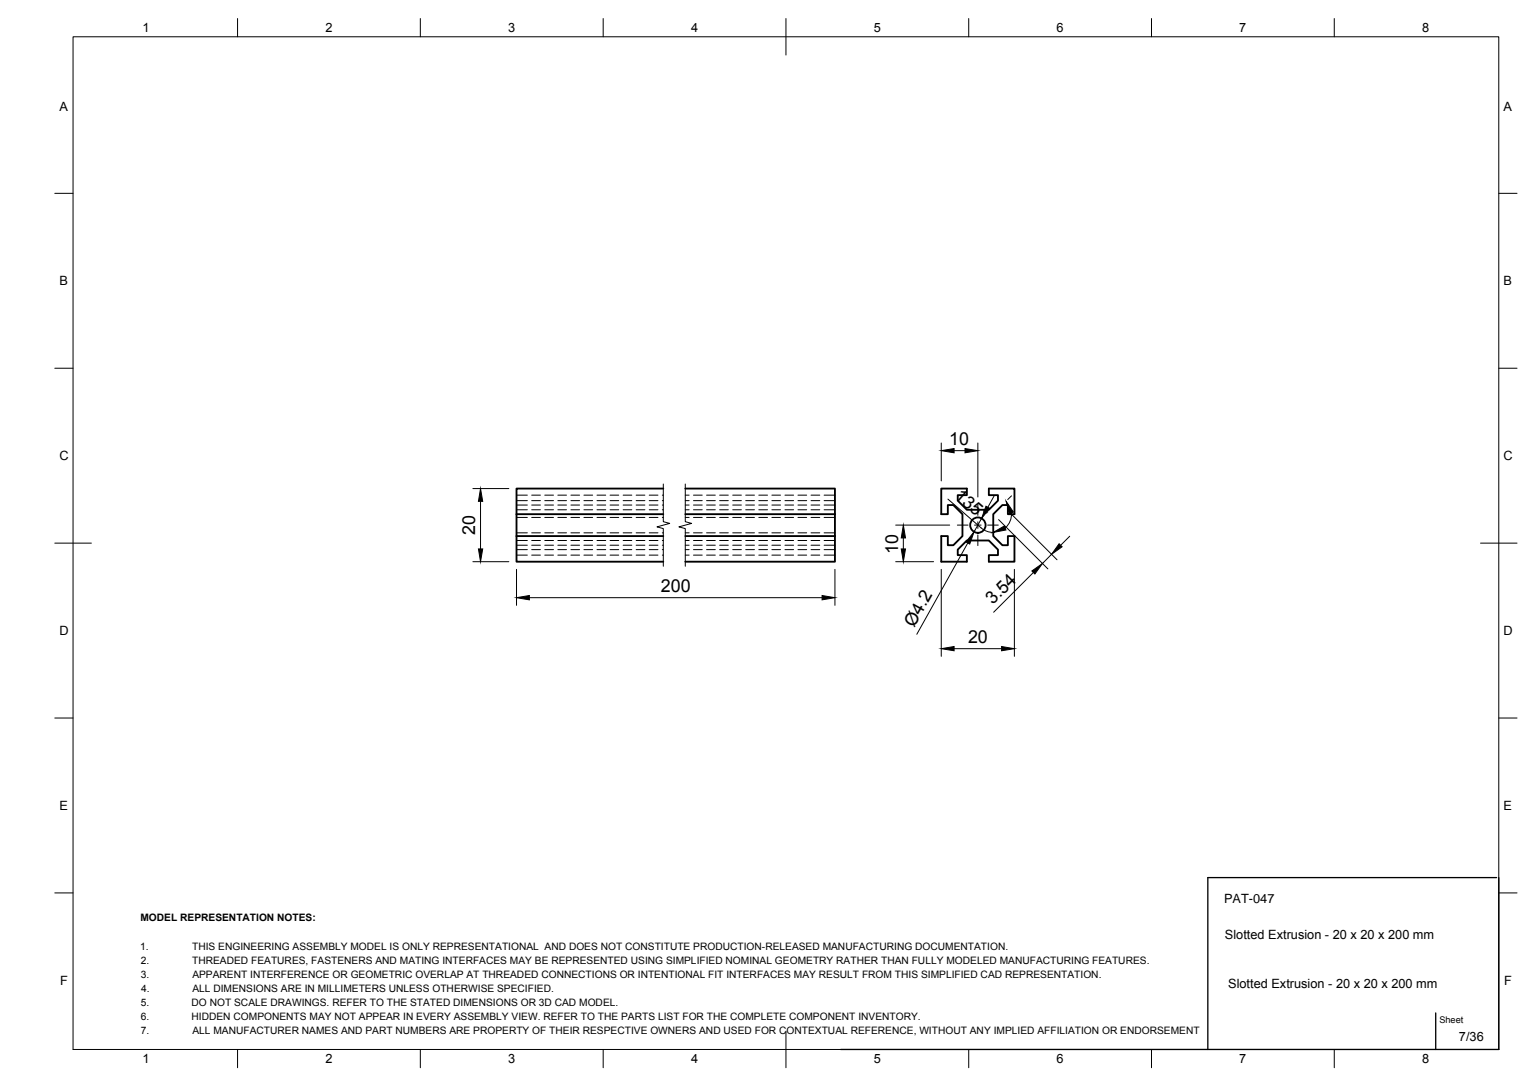
ISO-10303-21;
HEADER;
/* Generated by software containing ST-Developer
 * from STEP Tools, Inc. (www.steptools.com) 
 */

FILE_DESCRIPTION(
/* description */ ('Gravity roller conveyor section'),
/* implementation_level */ '2;1');

FILE_NAME(
/* name */ 'Slotted Extrusion - 20 x 20 x 200 mm.step',
/* time_stamp */ '2026-11-02T07:43:02-08:00',
/* author */ (''),
/* organization */ (''),
/* preprocessor_version */ 'ST-DEVELOPER v20.2',
/* originating_system */ 'Autodesk Translation Framework v15.17.0.0',
/* authorisation */ '');

FILE_SCHEMA (('AUTOMOTIVE_DESIGN { 1 0 10303 214 3 1 1 }'));
ENDSEC;

DATA;
#10=MECHANICAL_DESIGN_GEOMETRIC_PRESENTATION_REPRESENTATION('',(#532),#13821);
#464=SHAPE_REPRESENTATION_RELATIONSHIP('SRR','None',#14001,#498);
#498=ADVANCED_BREP_SHAPE_REPRESENTATION('',(#574),#13788);
#532=STYLED_ITEM('',(#14192),#574);
#574=MANIFOLD_SOLID_BREP('Body1',#7630);
#627=FACE_BOUND('',#1598,.T.);
#628=FACE_BOUND('',#1600,.T.);
#800=PLANE('',#8178);
#801=PLANE('',#8179);
#802=PLANE('',#8180);
#803=PLANE('',#8181);
#804=PLANE('',#8182);
#805=PLANE('',#8183);
#806=PLANE('',#8184);
#807=PLANE('',#8185);
#808=PLANE('',#8186);
#809=PLANE('',#8187);
#810=PLANE('',#8188);
#811=PLANE('',#8189);
#812=PLANE('',#8190);
#813=PLANE('',#8191);
#814=PLANE('',#8192);
#815=PLANE('',#8193);
#816=PLANE('',#8194);
#817=PLANE('',#8195);
#818=PLANE('',#8196);
#819=PLANE('',#8197);
#820=PLANE('',#8198);
#821=PLANE('',#8199);
#822=PLANE('',#8200);
#823=PLANE('',#8201);
#824=PLANE('',#8202);
#825=PLANE('',#8203);
#826=PLANE('',#8204);
#827=PLANE('',#8205);
#828=PLANE('',#8206);
#829=PLANE('',#8207);
#830=PLANE('',#8208);
#831=PLANE('',#8209);
#832=PLANE('',#8210);
#833=PLANE('',#8211);
#834=PLANE('',#8212);
#835=PLANE('',#8213);
#836=PLANE('',#8217);
#837=PLANE('',#8218);
#838=PLANE('',#8219);
#839=PLANE('',#8220);
#840=PLANE('',#8221);
#841=PLANE('',#8222);
#842=PLANE('',#8223);
#843=PLANE('',#8224);
#844=PLANE('',#8225);
#845=PLANE('',#8226);
#1115=FACE_OUTER_BOUND('',#1552,.T.);
#1116=FACE_OUTER_BOUND('',#1553,.T.);
#1117=FACE_OUTER_BOUND('',#1554,.T.);
#1118=FACE_OUTER_BOUND('',#1555,.T.);
#1119=FACE_OUTER_BOUND('',#1556,.T.);
#1120=FACE_OUTER_BOUND('',#1557,.T.);
#1121=FACE_OUTER_BOUND('',#1558,.T.);
#1122=FACE_OUTER_BOUND('',#1559,.T.);
#1123=FACE_OUTER_BOUND('',#1560,.T.);
#1124=FACE_OUTER_BOUND('',#1561,.T.);
#1125=FACE_OUTER_BOUND('',#1562,.T.);
#1126=FACE_OUTER_BOUND('',#1563,.T.);
#1127=FACE_OUTER_BOUND('',#1564,.T.);
#1128=FACE_OUTER_BOUND('',#1565,.T.);
#1129=FACE_OUTER_BOUND('',#1566,.T.);
#1130=FACE_OUTER_BOUND('',#1567,.T.);
#1131=FACE_OUTER_BOUND('',#1568,.T.);
#1132=FACE_OUTER_BOUND('',#1569,.T.);
#1133=FACE_OUTER_BOUND('',#1570,.T.);
#1134=FACE_OUTER_BOUND('',#1571,.T.);
#1135=FACE_OUTER_BOUND('',#1572,.T.);
#1136=FACE_OUTER_BOUND('',#1573,.T.);
#1137=FACE_OUTER_BOUND('',#1574,.T.);
#1138=FACE_OUTER_BOUND('',#1575,.T.);
#1139=FACE_OUTER_BOUND('',#1576,.T.);
#1140=FACE_OUTER_BOUND('',#1577,.T.);
#1141=FACE_OUTER_BOUND('',#1578,.T.);
#1142=FACE_OUTER_BOUND('',#1579,.T.);
#1143=FACE_OUTER_BOUND('',#1580,.T.);
#1144=FACE_OUTER_BOUND('',#1581,.T.);
#1145=FACE_OUTER_BOUND('',#1582,.T.);
#1146=FACE_OUTER_BOUND('',#1583,.T.);
#1147=FACE_OUTER_BOUND('',#1584,.T.);
#1148=FACE_OUTER_BOUND('',#1585,.T.);
#1149=FACE_OUTER_BOUND('',#1586,.T.);
#1150=FACE_OUTER_BOUND('',#1587,.T.);
#1151=FACE_OUTER_BOUND('',#1588,.T.);
#1152=FACE_OUTER_BOUND('',#1589,.T.);
#1153=FACE_OUTER_BOUND('',#1590,.T.);
#1154=FACE_OUTER_BOUND('',#1591,.T.);
#1155=FACE_OUTER_BOUND('',#1592,.T.);
#1156=FACE_OUTER_BOUND('',#1593,.T.);
#1157=FACE_OUTER_BOUND('',#1594,.T.);
#1158=FACE_OUTER_BOUND('',#1595,.T.);
#1159=FACE_OUTER_BOUND('',#1596,.T.);
#1160=FACE_OUTER_BOUND('',#1597,.T.);
#1161=FACE_OUTER_BOUND('',#1599,.T.);
#1552=EDGE_LOOP('',(#5830,#5831,#5832,#5833));
#1553=EDGE_LOOP('',(#5834,#5835,#5836,#5837));
#1554=EDGE_LOOP('',(#5838,#5839,#5840,#5841));
#1555=EDGE_LOOP('',(#5842,#5843,#5844,#5845));
#1556=EDGE_LOOP('',(#5846,#5847,#5848,#5849));
#1557=EDGE_LOOP('',(#5850,#5851,#5852,#5853));
#1558=EDGE_LOOP('',(#5854,#5855,#5856,#5857));
#1559=EDGE_LOOP('',(#5858,#5859,#5860,#5861));
#1560=EDGE_LOOP('',(#5862,#5863,#5864,#5865));
#1561=EDGE_LOOP('',(#5866,#5867,#5868,#5869));
#1562=EDGE_LOOP('',(#5870,#5871,#5872,#5873));
#1563=EDGE_LOOP('',(#5874,#5875,#5876,#5877));
#1564=EDGE_LOOP('',(#5878,#5879,#5880,#5881));
#1565=EDGE_LOOP('',(#5882,#5883,#5884,#5885));
#1566=EDGE_LOOP('',(#5886,#5887,#5888,#5889));
#1567=EDGE_LOOP('',(#5890,#5891,#5892,#5893));
#1568=EDGE_LOOP('',(#5894,#5895,#5896,#5897));
#1569=EDGE_LOOP('',(#5898,#5899,#5900,#5901));
#1570=EDGE_LOOP('',(#5902,#5903,#5904,#5905));
#1571=EDGE_LOOP('',(#5906,#5907,#5908,#5909));
#1572=EDGE_LOOP('',(#5910,#5911,#5912,#5913));
#1573=EDGE_LOOP('',(#5914,#5915,#5916,#5917));
#1574=EDGE_LOOP('',(#5918,#5919,#5920,#5921));
#1575=EDGE_LOOP('',(#5922,#5923,#5924,#5925));
#1576=EDGE_LOOP('',(#5926,#5927,#5928,#5929));
#1577=EDGE_LOOP('',(#5930,#5931,#5932,#5933));
#1578=EDGE_LOOP('',(#5934,#5935,#5936,#5937));
#1579=EDGE_LOOP('',(#5938,#5939,#5940,#5941));
#1580=EDGE_LOOP('',(#5942,#5943,#5944,#5945));
#1581=EDGE_LOOP('',(#5946,#5947,#5948,#5949));
#1582=EDGE_LOOP('',(#5950,#5951,#5952,#5953));
#1583=EDGE_LOOP('',(#5954,#5955,#5956,#5957));
#1584=EDGE_LOOP('',(#5958,#5959,#5960,#5961));
#1585=EDGE_LOOP('',(#5962,#5963,#5964,#5965));
#1586=EDGE_LOOP('',(#5966,#5967,#5968,#5969));
#1587=EDGE_LOOP('',(#5970,#5971,#5972,#5973));
#1588=EDGE_LOOP('',(#5974,#5975,#5976,#5977));
#1589=EDGE_LOOP('',(#5978,#5979,#5980,#5981));
#1590=EDGE_LOOP('',(#5982,#5983,#5984,#5985));
#1591=EDGE_LOOP('',(#5986,#5987,#5988,#5989));
#1592=EDGE_LOOP('',(#5990,#5991,#5992,#5993));
#1593=EDGE_LOOP('',(#5994,#5995,#5996,#5997));
#1594=EDGE_LOOP('',(#5998,#5999,#6000,#6001));
#1595=EDGE_LOOP('',(#6002,#6003,#6004,#6005));
#1596=EDGE_LOOP('',(#6006,#6007,#6008,#6009));
#1597=EDGE_LOOP('',(#6010,#6011,#6012,#6013,#6014,#6015,#6016,#6017,#6018,
#6019,#6020,#6021,#6022,#6023,#6024,#6025,#6026,#6027,#6028,#6029,#6030,
#6031,#6032,#6033,#6034,#6035,#6036,#6037,#6038,#6039,#6040,#6041,#6042,
#6043,#6044,#6045,#6046,#6047,#6048,#6049,#6050,#6051,#6052,#6053));
#1598=EDGE_LOOP('',(#6054));
#1599=EDGE_LOOP('',(#6055,#6056,#6057,#6058,#6059,#6060,#6061,#6062,#6063,
#6064,#6065,#6066,#6067,#6068,#6069,#6070,#6071,#6072,#6073,#6074,#6075,
#6076,#6077,#6078,#6079,#6080,#6081,#6082,#6083,#6084,#6085,#6086,#6087,
#6088,#6089,#6090,#6091,#6092,#6093,#6094,#6095,#6096,#6097,#6098));
#1600=EDGE_LOOP('',(#6099));
#2226=LINE('',#11884,#2944);
#2227=LINE('',#11886,#2945);
#2228=LINE('',#11888,#2946);
#2229=LINE('',#11889,#2947);
#2230=LINE('',#11892,#2948);
#2231=LINE('',#11894,#2949);
#2232=LINE('',#11895,#2950);
#2233=LINE('',#11898,#2951);
#2234=LINE('',#11900,#2952);
#2235=LINE('',#11901,#2953);
#2236=LINE('',#11904,#2954);
#2237=LINE('',#11906,#2955);
#2238=LINE('',#11907,#2956);
#2239=LINE('',#11910,#2957);
#2240=LINE('',#11912,#2958);
#2241=LINE('',#11913,#2959);
#2242=LINE('',#11916,#2960);
#2243=LINE('',#11918,#2961);
#2244=LINE('',#11919,#2962);
#2245=LINE('',#11922,#2963);
#2246=LINE('',#11924,#2964);
#2247=LINE('',#11925,#2965);
#2248=LINE('',#11928,#2966);
#2249=LINE('',#11930,#2967);
#2250=LINE('',#11931,#2968);
#2251=LINE('',#11934,#2969);
#2252=LINE('',#11936,#2970);
#2253=LINE('',#11937,#2971);
#2254=LINE('',#11941,#2972);
#2255=LINE('',#11943,#2973);
#2256=LINE('',#11945,#2974);
#2257=LINE('',#11946,#2975);
#2258=LINE('',#11949,#2976);
#2259=LINE('',#11951,#2977);
#2260=LINE('',#11952,#2978);
#2261=LINE('',#11955,#2979);
#2262=LINE('',#11957,#2980);
#2263=LINE('',#11958,#2981);
#2264=LINE('',#11961,#2982);
#2265=LINE('',#11963,#2983);
#2266=LINE('',#11964,#2984);
#2267=LINE('',#11967,#2985);
#2268=LINE('',#11969,#2986);
#2269=LINE('',#11970,#2987);
#2270=LINE('',#11973,#2988);
#2271=LINE('',#11975,#2989);
#2272=LINE('',#11976,#2990);
#2273=LINE('',#11979,#2991);
#2274=LINE('',#11981,#2992);
#2275=LINE('',#11982,#2993);
#2276=LINE('',#11985,#2994);
#2277=LINE('',#11987,#2995);
#2278=LINE('',#11988,#2996);
#2279=LINE('',#11991,#2997);
#2280=LINE('',#11993,#2998);
#2281=LINE('',#11994,#2999);
#2282=LINE('',#11998,#3000);
#2283=LINE('',#12000,#3001);
#2284=LINE('',#12002,#3002);
#2285=LINE('',#12003,#3003);
#2286=LINE('',#12006,#3004);
#2287=LINE('',#12008,#3005);
#2288=LINE('',#12009,#3006);
#2289=LINE('',#12012,#3007);
#2290=LINE('',#12014,#3008);
#2291=LINE('',#12015,#3009);
#2292=LINE('',#12018,#3010);
#2293=LINE('',#12020,#3011);
#2294=LINE('',#12021,#3012);
#2295=LINE('',#12024,#3013);
#2296=LINE('',#12026,#3014);
#2297=LINE('',#12027,#3015);
#2298=LINE('',#12030,#3016);
#2299=LINE('',#12032,#3017);
#2300=LINE('',#12033,#3018);
#2301=LINE('',#12036,#3019);
#2302=LINE('',#12038,#3020);
#2303=LINE('',#12039,#3021);
#2304=LINE('',#12042,#3022);
#2305=LINE('',#12044,#3023);
#2306=LINE('',#12045,#3024);
#2307=LINE('',#12048,#3025);
#2308=LINE('',#12050,#3026);
#2309=LINE('',#12051,#3027);
#2310=LINE('',#12055,#3028);
#2311=LINE('',#12057,#3029);
#2312=LINE('',#12059,#3030);
#2313=LINE('',#12060,#3031);
#2314=LINE('',#12063,#3032);
#2315=LINE('',#12065,#3033);
#2316=LINE('',#12066,#3034);
#2317=LINE('',#12069,#3035);
#2318=LINE('',#12071,#3036);
#2319=LINE('',#12072,#3037);
#2320=LINE('',#12075,#3038);
#2321=LINE('',#12077,#3039);
#2322=LINE('',#12078,#3040);
#2323=LINE('',#12081,#3041);
#2324=LINE('',#12083,#3042);
#2325=LINE('',#12084,#3043);
#2326=LINE('',#12087,#3044);
#2327=LINE('',#12089,#3045);
#2328=LINE('',#12090,#3046);
#2329=LINE('',#12093,#3047);
#2330=LINE('',#12095,#3048);
#2331=LINE('',#12096,#3049);
#2332=LINE('',#12099,#3050);
#2333=LINE('',#12101,#3051);
#2334=LINE('',#12102,#3052);
#2335=LINE('',#12105,#3053);
#2336=LINE('',#12107,#3054);
#2337=LINE('',#12108,#3055);
#2338=LINE('',#12113,#3056);
#2339=LINE('',#12117,#3057);
#2340=LINE('',#12119,#3058);
#2341=LINE('',#12120,#3059);
#2342=LINE('',#12123,#3060);
#2343=LINE('',#12125,#3061);
#2344=LINE('',#12126,#3062);
#2345=LINE('',#12128,#3063);
#2346=LINE('',#12129,#3064);
#2347=LINE('',#12132,#3065);
#2348=LINE('',#12134,#3066);
#2349=LINE('',#12135,#3067);
#2350=LINE('',#12137,#3068);
#2351=LINE('',#12138,#3069);
#2352=LINE('',#12141,#3070);
#2353=LINE('',#12143,#3071);
#2354=LINE('',#12144,#3072);
#2355=LINE('',#12146,#3073);
#2356=LINE('',#12147,#3074);
#2357=LINE('',#12149,#3075);
#2358=LINE('',#12150,#3076);
#2944=VECTOR('',#9367,1.);
#2945=VECTOR('',#9368,1.);
#2946=VECTOR('',#9369,1.);
#2947=VECTOR('',#9370,1.);
#2948=VECTOR('',#9373,1.);
#2949=VECTOR('',#9374,1.);
#2950=VECTOR('',#9375,1.);
#2951=VECTOR('',#9378,1.);
#2952=VECTOR('',#9379,1.);
#2953=VECTOR('',#9380,1.);
#2954=VECTOR('',#9383,1.);
#2955=VECTOR('',#9384,1.);
#2956=VECTOR('',#9385,1.);
#2957=VECTOR('',#9388,1.);
#2958=VECTOR('',#9389,1.);
#2959=VECTOR('',#9390,1.);
#2960=VECTOR('',#9393,1.);
#2961=VECTOR('',#9394,1.);
#2962=VECTOR('',#9395,1.);
#2963=VECTOR('',#9398,1.);
#2964=VECTOR('',#9399,1.);
#2965=VECTOR('',#9400,1.);
#2966=VECTOR('',#9403,1.);
#2967=VECTOR('',#9404,1.);
#2968=VECTOR('',#9405,1.);
#2969=VECTOR('',#9408,1.);
#2970=VECTOR('',#9409,1.);
#2971=VECTOR('',#9410,1.);
#2972=VECTOR('',#9413,1.);
#2973=VECTOR('',#9414,1.);
#2974=VECTOR('',#9415,1.);
#2975=VECTOR('',#9416,1.);
#2976=VECTOR('',#9419,1.);
#2977=VECTOR('',#9420,1.);
#2978=VECTOR('',#9421,1.);
#2979=VECTOR('',#9424,1.);
#2980=VECTOR('',#9425,1.);
#2981=VECTOR('',#9426,1.);
#2982=VECTOR('',#9429,1.);
#2983=VECTOR('',#9430,1.);
#2984=VECTOR('',#9431,1.);
#2985=VECTOR('',#9434,1.);
#2986=VECTOR('',#9435,1.);
#2987=VECTOR('',#9436,1.);
#2988=VECTOR('',#9439,1.);
#2989=VECTOR('',#9440,1.);
#2990=VECTOR('',#9441,1.);
#2991=VECTOR('',#9444,1.);
#2992=VECTOR('',#9445,1.);
#2993=VECTOR('',#9446,1.);
#2994=VECTOR('',#9449,1.);
#2995=VECTOR('',#9450,1.);
#2996=VECTOR('',#9451,1.);
#2997=VECTOR('',#9454,1.);
#2998=VECTOR('',#9455,1.);
#2999=VECTOR('',#9456,1.);
#3000=VECTOR('',#9459,1.);
#3001=VECTOR('',#9460,1.);
#3002=VECTOR('',#9461,1.);
#3003=VECTOR('',#9462,1.);
#3004=VECTOR('',#9465,1.);
#3005=VECTOR('',#9466,1.);
#3006=VECTOR('',#9467,1.);
#3007=VECTOR('',#9470,1.);
#3008=VECTOR('',#9471,1.);
#3009=VECTOR('',#9472,1.);
#3010=VECTOR('',#9475,1.);
#3011=VECTOR('',#9476,1.);
#3012=VECTOR('',#9477,1.);
#3013=VECTOR('',#9480,1.);
#3014=VECTOR('',#9481,1.);
#3015=VECTOR('',#9482,1.);
#3016=VECTOR('',#9485,1.);
#3017=VECTOR('',#9486,1.);
#3018=VECTOR('',#9487,1.);
#3019=VECTOR('',#9490,1.);
#3020=VECTOR('',#9491,1.);
#3021=VECTOR('',#9492,1.);
#3022=VECTOR('',#9495,1.);
#3023=VECTOR('',#9496,1.);
#3024=VECTOR('',#9497,1.);
#3025=VECTOR('',#9500,1.);
#3026=VECTOR('',#9501,1.);
#3027=VECTOR('',#9502,1.);
#3028=VECTOR('',#9505,1.);
#3029=VECTOR('',#9506,1.);
#3030=VECTOR('',#9507,1.);
#3031=VECTOR('',#9508,1.);
#3032=VECTOR('',#9511,1.);
#3033=VECTOR('',#9512,1.);
#3034=VECTOR('',#9513,1.);
#3035=VECTOR('',#9516,1.);
#3036=VECTOR('',#9517,1.);
#3037=VECTOR('',#9518,1.);
#3038=VECTOR('',#9521,1.);
#3039=VECTOR('',#9522,1.);
#3040=VECTOR('',#9523,1.);
#3041=VECTOR('',#9526,1.);
#3042=VECTOR('',#9527,1.);
#3043=VECTOR('',#9528,1.);
#3044=VECTOR('',#9531,1.);
#3045=VECTOR('',#9532,1.);
#3046=VECTOR('',#9533,1.);
#3047=VECTOR('',#9536,1.);
#3048=VECTOR('',#9537,1.);
#3049=VECTOR('',#9538,1.);
#3050=VECTOR('',#9541,1.);
#3051=VECTOR('',#9542,1.);
#3052=VECTOR('',#9543,1.);
#3053=VECTOR('',#9546,1.);
#3054=VECTOR('',#9547,1.);
#3055=VECTOR('',#9548,1.);
#3056=VECTOR('',#9553,0.21);
#3057=VECTOR('',#9558,1.);
#3058=VECTOR('',#9559,1.);
#3059=VECTOR('',#9560,1.);
#3060=VECTOR('',#9563,1.);
#3061=VECTOR('',#9564,1.);
#3062=VECTOR('',#9565,1.);
#3063=VECTOR('',#9568,1.);
#3064=VECTOR('',#9569,1.);
#3065=VECTOR('',#9572,1.);
#3066=VECTOR('',#9573,1.);
#3067=VECTOR('',#9574,1.);
#3068=VECTOR('',#9577,1.);
#3069=VECTOR('',#9578,1.);
#3070=VECTOR('',#9581,1.);
#3071=VECTOR('',#9582,1.);
#3072=VECTOR('',#9583,1.);
#3073=VECTOR('',#9586,1.);
#3074=VECTOR('',#9587,1.);
#3075=VECTOR('',#9590,1.);
#3076=VECTOR('',#9591,1.);
#3390=CIRCLE('',#8215,0.21);
#3391=CIRCLE('',#8216,0.21);
#3800=VERTEX_POINT('',#11882);
#3801=VERTEX_POINT('',#11883);
#3802=VERTEX_POINT('',#11885);
#3803=VERTEX_POINT('',#11887);
#3804=VERTEX_POINT('',#11891);
#3805=VERTEX_POINT('',#11893);
#3806=VERTEX_POINT('',#11897);
#3807=VERTEX_POINT('',#11899);
#3808=VERTEX_POINT('',#11903);
#3809=VERTEX_POINT('',#11905);
#3810=VERTEX_POINT('',#11909);
#3811=VERTEX_POINT('',#11911);
#3812=VERTEX_POINT('',#11915);
#3813=VERTEX_POINT('',#11917);
#3814=VERTEX_POINT('',#11921);
#3815=VERTEX_POINT('',#11923);
#3816=VERTEX_POINT('',#11927);
#3817=VERTEX_POINT('',#11929);
#3818=VERTEX_POINT('',#11933);
#3819=VERTEX_POINT('',#11935);
#3820=VERTEX_POINT('',#11939);
#3821=VERTEX_POINT('',#11940);
#3822=VERTEX_POINT('',#11942);
#3823=VERTEX_POINT('',#11944);
#3824=VERTEX_POINT('',#11948);
#3825=VERTEX_POINT('',#11950);
#3826=VERTEX_POINT('',#11954);
#3827=VERTEX_POINT('',#11956);
#3828=VERTEX_POINT('',#11960);
#3829=VERTEX_POINT('',#11962);
#3830=VERTEX_POINT('',#11966);
#3831=VERTEX_POINT('',#11968);
#3832=VERTEX_POINT('',#11972);
#3833=VERTEX_POINT('',#11974);
#3834=VERTEX_POINT('',#11978);
#3835=VERTEX_POINT('',#11980);
#3836=VERTEX_POINT('',#11984);
#3837=VERTEX_POINT('',#11986);
#3838=VERTEX_POINT('',#11990);
#3839=VERTEX_POINT('',#11992);
#3840=VERTEX_POINT('',#11996);
#3841=VERTEX_POINT('',#11997);
#3842=VERTEX_POINT('',#11999);
#3843=VERTEX_POINT('',#12001);
#3844=VERTEX_POINT('',#12005);
#3845=VERTEX_POINT('',#12007);
#3846=VERTEX_POINT('',#12011);
#3847=VERTEX_POINT('',#12013);
#3848=VERTEX_POINT('',#12017);
#3849=VERTEX_POINT('',#12019);
#3850=VERTEX_POINT('',#12023);
#3851=VERTEX_POINT('',#12025);
#3852=VERTEX_POINT('',#12029);
#3853=VERTEX_POINT('',#12031);
#3854=VERTEX_POINT('',#12035);
#3855=VERTEX_POINT('',#12037);
#3856=VERTEX_POINT('',#12041);
#3857=VERTEX_POINT('',#12043);
#3858=VERTEX_POINT('',#12047);
#3859=VERTEX_POINT('',#12049);
#3860=VERTEX_POINT('',#12053);
#3861=VERTEX_POINT('',#12054);
#3862=VERTEX_POINT('',#12056);
#3863=VERTEX_POINT('',#12058);
#3864=VERTEX_POINT('',#12062);
#3865=VERTEX_POINT('',#12064);
#3866=VERTEX_POINT('',#12068);
#3867=VERTEX_POINT('',#12070);
#3868=VERTEX_POINT('',#12074);
#3869=VERTEX_POINT('',#12076);
#3870=VERTEX_POINT('',#12080);
#3871=VERTEX_POINT('',#12082);
#3872=VERTEX_POINT('',#12086);
#3873=VERTEX_POINT('',#12088);
#3874=VERTEX_POINT('',#12092);
#3875=VERTEX_POINT('',#12094);
#3876=VERTEX_POINT('',#12098);
#3877=VERTEX_POINT('',#12100);
#3878=VERTEX_POINT('',#12104);
#3879=VERTEX_POINT('',#12106);
#3880=VERTEX_POINT('',#12110);
#3881=VERTEX_POINT('',#12112);
#3882=VERTEX_POINT('',#12116);
#3883=VERTEX_POINT('',#12118);
#3884=VERTEX_POINT('',#12122);
#3885=VERTEX_POINT('',#12124);
#3886=VERTEX_POINT('',#12131);
#3887=VERTEX_POINT('',#12133);
#3888=VERTEX_POINT('',#12140);
#3889=VERTEX_POINT('',#12142);
#4552=EDGE_CURVE('',#3800,#3801,#2226,.T.);
#4553=EDGE_CURVE('',#3800,#3802,#2227,.T.);
#4554=EDGE_CURVE('',#3803,#3802,#2228,.T.);
#4555=EDGE_CURVE('',#3801,#3803,#2229,.T.);
#4556=EDGE_CURVE('',#3804,#3800,#2230,.T.);
#4557=EDGE_CURVE('',#3804,#3805,#2231,.T.);
#4558=EDGE_CURVE('',#3802,#3805,#2232,.T.);
#4559=EDGE_CURVE('',#3806,#3804,#2233,.T.);
#4560=EDGE_CURVE('',#3806,#3807,#2234,.T.);
#4561=EDGE_CURVE('',#3805,#3807,#2235,.T.);
#4562=EDGE_CURVE('',#3808,#3806,#2236,.T.);
#4563=EDGE_CURVE('',#3808,#3809,#2237,.T.);
#4564=EDGE_CURVE('',#3807,#3809,#2238,.T.);
#4565=EDGE_CURVE('',#3810,#3808,#2239,.T.);
#4566=EDGE_CURVE('',#3810,#3811,#2240,.T.);
#4567=EDGE_CURVE('',#3809,#3811,#2241,.T.);
#4568=EDGE_CURVE('',#3812,#3810,#2242,.T.);
#4569=EDGE_CURVE('',#3812,#3813,#2243,.T.);
#4570=EDGE_CURVE('',#3811,#3813,#2244,.T.);
#4571=EDGE_CURVE('',#3814,#3812,#2245,.T.);
#4572=EDGE_CURVE('',#3814,#3815,#2246,.T.);
#4573=EDGE_CURVE('',#3813,#3815,#2247,.T.);
#4574=EDGE_CURVE('',#3816,#3814,#2248,.T.);
#4575=EDGE_CURVE('',#3816,#3817,#2249,.T.);
#4576=EDGE_CURVE('',#3815,#3817,#2250,.T.);
#4577=EDGE_CURVE('',#3818,#3816,#2251,.T.);
#4578=EDGE_CURVE('',#3819,#3818,#2252,.T.);
#4579=EDGE_CURVE('',#3817,#3819,#2253,.T.);
#4580=EDGE_CURVE('',#3820,#3821,#2254,.T.);
#4581=EDGE_CURVE('',#3820,#3822,#2255,.T.);
#4582=EDGE_CURVE('',#3823,#3822,#2256,.T.);
#4583=EDGE_CURVE('',#3821,#3823,#2257,.T.);
#4584=EDGE_CURVE('',#3824,#3820,#2258,.T.);
#4585=EDGE_CURVE('',#3824,#3825,#2259,.T.);
#4586=EDGE_CURVE('',#3822,#3825,#2260,.T.);
#4587=EDGE_CURVE('',#3826,#3824,#2261,.T.);
#4588=EDGE_CURVE('',#3826,#3827,#2262,.T.);
#4589=EDGE_CURVE('',#3825,#3827,#2263,.T.);
#4590=EDGE_CURVE('',#3828,#3826,#2264,.T.);
#4591=EDGE_CURVE('',#3828,#3829,#2265,.T.);
#4592=EDGE_CURVE('',#3827,#3829,#2266,.T.);
#4593=EDGE_CURVE('',#3830,#3828,#2267,.T.);
#4594=EDGE_CURVE('',#3830,#3831,#2268,.T.);
#4595=EDGE_CURVE('',#3829,#3831,#2269,.T.);
#4596=EDGE_CURVE('',#3832,#3830,#2270,.T.);
#4597=EDGE_CURVE('',#3832,#3833,#2271,.T.);
#4598=EDGE_CURVE('',#3831,#3833,#2272,.T.);
#4599=EDGE_CURVE('',#3834,#3832,#2273,.T.);
#4600=EDGE_CURVE('',#3834,#3835,#2274,.T.);
#4601=EDGE_CURVE('',#3833,#3835,#2275,.T.);
#4602=EDGE_CURVE('',#3836,#3834,#2276,.T.);
#4603=EDGE_CURVE('',#3836,#3837,#2277,.T.);
#4604=EDGE_CURVE('',#3835,#3837,#2278,.T.);
#4605=EDGE_CURVE('',#3838,#3836,#2279,.T.);
#4606=EDGE_CURVE('',#3839,#3838,#2280,.T.);
#4607=EDGE_CURVE('',#3837,#3839,#2281,.T.);
#4608=EDGE_CURVE('',#3840,#3841,#2282,.T.);
#4609=EDGE_CURVE('',#3840,#3842,#2283,.T.);
#4610=EDGE_CURVE('',#3843,#3842,#2284,.T.);
#4611=EDGE_CURVE('',#3841,#3843,#2285,.T.);
#4612=EDGE_CURVE('',#3844,#3840,#2286,.T.);
#4613=EDGE_CURVE('',#3844,#3845,#2287,.T.);
#4614=EDGE_CURVE('',#3842,#3845,#2288,.T.);
#4615=EDGE_CURVE('',#3846,#3844,#2289,.T.);
#4616=EDGE_CURVE('',#3846,#3847,#2290,.T.);
#4617=EDGE_CURVE('',#3845,#3847,#2291,.T.);
#4618=EDGE_CURVE('',#3848,#3846,#2292,.T.);
#4619=EDGE_CURVE('',#3848,#3849,#2293,.T.);
#4620=EDGE_CURVE('',#3847,#3849,#2294,.T.);
#4621=EDGE_CURVE('',#3850,#3848,#2295,.T.);
#4622=EDGE_CURVE('',#3850,#3851,#2296,.T.);
#4623=EDGE_CURVE('',#3849,#3851,#2297,.T.);
#4624=EDGE_CURVE('',#3852,#3850,#2298,.T.);
#4625=EDGE_CURVE('',#3852,#3853,#2299,.T.);
#4626=EDGE_CURVE('',#3851,#3853,#2300,.T.);
#4627=EDGE_CURVE('',#3854,#3852,#2301,.T.);
#4628=EDGE_CURVE('',#3854,#3855,#2302,.T.);
#4629=EDGE_CURVE('',#3853,#3855,#2303,.T.);
#4630=EDGE_CURVE('',#3856,#3854,#2304,.T.);
#4631=EDGE_CURVE('',#3856,#3857,#2305,.T.);
#4632=EDGE_CURVE('',#3855,#3857,#2306,.T.);
#4633=EDGE_CURVE('',#3858,#3856,#2307,.T.);
#4634=EDGE_CURVE('',#3859,#3858,#2308,.T.);
#4635=EDGE_CURVE('',#3857,#3859,#2309,.T.);
#4636=EDGE_CURVE('',#3860,#3861,#2310,.T.);
#4637=EDGE_CURVE('',#3860,#3862,#2311,.T.);
#4638=EDGE_CURVE('',#3863,#3862,#2312,.T.);
#4639=EDGE_CURVE('',#3861,#3863,#2313,.T.);
#4640=EDGE_CURVE('',#3864,#3860,#2314,.T.);
#4641=EDGE_CURVE('',#3864,#3865,#2315,.T.);
#4642=EDGE_CURVE('',#3862,#3865,#2316,.T.);
#4643=EDGE_CURVE('',#3866,#3864,#2317,.T.);
#4644=EDGE_CURVE('',#3866,#3867,#2318,.T.);
#4645=EDGE_CURVE('',#3865,#3867,#2319,.T.);
#4646=EDGE_CURVE('',#3868,#3866,#2320,.T.);
#4647=EDGE_CURVE('',#3868,#3869,#2321,.T.);
#4648=EDGE_CURVE('',#3867,#3869,#2322,.T.);
#4649=EDGE_CURVE('',#3870,#3868,#2323,.T.);
#4650=EDGE_CURVE('',#3870,#3871,#2324,.T.);
#4651=EDGE_CURVE('',#3869,#3871,#2325,.T.);
#4652=EDGE_CURVE('',#3872,#3870,#2326,.T.);
#4653=EDGE_CURVE('',#3872,#3873,#2327,.T.);
#4654=EDGE_CURVE('',#3871,#3873,#2328,.T.);
#4655=EDGE_CURVE('',#3874,#3872,#2329,.T.);
#4656=EDGE_CURVE('',#3874,#3875,#2330,.T.);
#4657=EDGE_CURVE('',#3873,#3875,#2331,.T.);
#4658=EDGE_CURVE('',#3876,#3874,#2332,.T.);
#4659=EDGE_CURVE('',#3876,#3877,#2333,.T.);
#4660=EDGE_CURVE('',#3875,#3877,#2334,.T.);
#4661=EDGE_CURVE('',#3878,#3876,#2335,.T.);
#4662=EDGE_CURVE('',#3879,#3878,#2336,.T.);
#4663=EDGE_CURVE('',#3877,#3879,#2337,.T.);
#4664=EDGE_CURVE('',#3880,#3880,#3390,.T.);
#4665=EDGE_CURVE('',#3880,#3881,#2338,.T.);
#4666=EDGE_CURVE('',#3881,#3881,#3391,.T.);
#4667=EDGE_CURVE('',#3818,#3882,#2339,.T.);
#4668=EDGE_CURVE('',#3882,#3883,#2340,.T.);
#4669=EDGE_CURVE('',#3819,#3883,#2341,.T.);
#4670=EDGE_CURVE('',#3884,#3803,#2342,.T.);
#4671=EDGE_CURVE('',#3885,#3884,#2343,.T.);
#4672=EDGE_CURVE('',#3885,#3801,#2344,.T.);
#4673=EDGE_CURVE('',#3838,#3885,#2345,.T.);
#4674=EDGE_CURVE('',#3839,#3884,#2346,.T.);
#4675=EDGE_CURVE('',#3886,#3823,#2347,.T.);
#4676=EDGE_CURVE('',#3887,#3886,#2348,.T.);
#4677=EDGE_CURVE('',#3887,#3821,#2349,.T.);
#4678=EDGE_CURVE('',#3858,#3887,#2350,.T.);
#4679=EDGE_CURVE('',#3859,#3886,#2351,.T.);
#4680=EDGE_CURVE('',#3888,#3843,#2352,.T.);
#4681=EDGE_CURVE('',#3889,#3888,#2353,.T.);
#4682=EDGE_CURVE('',#3889,#3841,#2354,.T.);
#4683=EDGE_CURVE('',#3878,#3889,#2355,.T.);
#4684=EDGE_CURVE('',#3879,#3888,#2356,.T.);
#4685=EDGE_CURVE('',#3883,#3863,#2357,.T.);
#4686=EDGE_CURVE('',#3882,#3861,#2358,.T.);
#5830=ORIENTED_EDGE('',*,*,#4552,.F.);
#5831=ORIENTED_EDGE('',*,*,#4553,.T.);
#5832=ORIENTED_EDGE('',*,*,#4554,.F.);
#5833=ORIENTED_EDGE('',*,*,#4555,.F.);
#5834=ORIENTED_EDGE('',*,*,#4556,.F.);
#5835=ORIENTED_EDGE('',*,*,#4557,.T.);
#5836=ORIENTED_EDGE('',*,*,#4558,.F.);
#5837=ORIENTED_EDGE('',*,*,#4553,.F.);
#5838=ORIENTED_EDGE('',*,*,#4559,.F.);
#5839=ORIENTED_EDGE('',*,*,#4560,.T.);
#5840=ORIENTED_EDGE('',*,*,#4561,.F.);
#5841=ORIENTED_EDGE('',*,*,#4557,.F.);
#5842=ORIENTED_EDGE('',*,*,#4562,.F.);
#5843=ORIENTED_EDGE('',*,*,#4563,.T.);
#5844=ORIENTED_EDGE('',*,*,#4564,.F.);
#5845=ORIENTED_EDGE('',*,*,#4560,.F.);
#5846=ORIENTED_EDGE('',*,*,#4565,.F.);
#5847=ORIENTED_EDGE('',*,*,#4566,.T.);
#5848=ORIENTED_EDGE('',*,*,#4567,.F.);
#5849=ORIENTED_EDGE('',*,*,#4563,.F.);
#5850=ORIENTED_EDGE('',*,*,#4568,.F.);
#5851=ORIENTED_EDGE('',*,*,#4569,.T.);
#5852=ORIENTED_EDGE('',*,*,#4570,.F.);
#5853=ORIENTED_EDGE('',*,*,#4566,.F.);
#5854=ORIENTED_EDGE('',*,*,#4571,.F.);
#5855=ORIENTED_EDGE('',*,*,#4572,.T.);
#5856=ORIENTED_EDGE('',*,*,#4573,.F.);
#5857=ORIENTED_EDGE('',*,*,#4569,.F.);
#5858=ORIENTED_EDGE('',*,*,#4574,.F.);
#5859=ORIENTED_EDGE('',*,*,#4575,.T.);
#5860=ORIENTED_EDGE('',*,*,#4576,.F.);
#5861=ORIENTED_EDGE('',*,*,#4572,.F.);
#5862=ORIENTED_EDGE('',*,*,#4577,.F.);
#5863=ORIENTED_EDGE('',*,*,#4578,.F.);
#5864=ORIENTED_EDGE('',*,*,#4579,.F.);
#5865=ORIENTED_EDGE('',*,*,#4575,.F.);
#5866=ORIENTED_EDGE('',*,*,#4580,.F.);
#5867=ORIENTED_EDGE('',*,*,#4581,.T.);
#5868=ORIENTED_EDGE('',*,*,#4582,.F.);
#5869=ORIENTED_EDGE('',*,*,#4583,.F.);
#5870=ORIENTED_EDGE('',*,*,#4584,.F.);
#5871=ORIENTED_EDGE('',*,*,#4585,.T.);
#5872=ORIENTED_EDGE('',*,*,#4586,.F.);
#5873=ORIENTED_EDGE('',*,*,#4581,.F.);
#5874=ORIENTED_EDGE('',*,*,#4587,.F.);
#5875=ORIENTED_EDGE('',*,*,#4588,.T.);
#5876=ORIENTED_EDGE('',*,*,#4589,.F.);
#5877=ORIENTED_EDGE('',*,*,#4585,.F.);
#5878=ORIENTED_EDGE('',*,*,#4590,.F.);
#5879=ORIENTED_EDGE('',*,*,#4591,.T.);
#5880=ORIENTED_EDGE('',*,*,#4592,.F.);
#5881=ORIENTED_EDGE('',*,*,#4588,.F.);
#5882=ORIENTED_EDGE('',*,*,#4593,.F.);
#5883=ORIENTED_EDGE('',*,*,#4594,.T.);
#5884=ORIENTED_EDGE('',*,*,#4595,.F.);
#5885=ORIENTED_EDGE('',*,*,#4591,.F.);
#5886=ORIENTED_EDGE('',*,*,#4596,.F.);
#5887=ORIENTED_EDGE('',*,*,#4597,.T.);
#5888=ORIENTED_EDGE('',*,*,#4598,.F.);
#5889=ORIENTED_EDGE('',*,*,#4594,.F.);
#5890=ORIENTED_EDGE('',*,*,#4599,.F.);
#5891=ORIENTED_EDGE('',*,*,#4600,.T.);
#5892=ORIENTED_EDGE('',*,*,#4601,.F.);
#5893=ORIENTED_EDGE('',*,*,#4597,.F.);
#5894=ORIENTED_EDGE('',*,*,#4602,.F.);
#5895=ORIENTED_EDGE('',*,*,#4603,.T.);
#5896=ORIENTED_EDGE('',*,*,#4604,.F.);
#5897=ORIENTED_EDGE('',*,*,#4600,.F.);
#5898=ORIENTED_EDGE('',*,*,#4605,.F.);
#5899=ORIENTED_EDGE('',*,*,#4606,.F.);
#5900=ORIENTED_EDGE('',*,*,#4607,.F.);
#5901=ORIENTED_EDGE('',*,*,#4603,.F.);
#5902=ORIENTED_EDGE('',*,*,#4608,.F.);
#5903=ORIENTED_EDGE('',*,*,#4609,.T.);
#5904=ORIENTED_EDGE('',*,*,#4610,.F.);
#5905=ORIENTED_EDGE('',*,*,#4611,.F.);
#5906=ORIENTED_EDGE('',*,*,#4612,.F.);
#5907=ORIENTED_EDGE('',*,*,#4613,.T.);
#5908=ORIENTED_EDGE('',*,*,#4614,.F.);
#5909=ORIENTED_EDGE('',*,*,#4609,.F.);
#5910=ORIENTED_EDGE('',*,*,#4615,.F.);
#5911=ORIENTED_EDGE('',*,*,#4616,.T.);
#5912=ORIENTED_EDGE('',*,*,#4617,.F.);
#5913=ORIENTED_EDGE('',*,*,#4613,.F.);
#5914=ORIENTED_EDGE('',*,*,#4618,.F.);
#5915=ORIENTED_EDGE('',*,*,#4619,.T.);
#5916=ORIENTED_EDGE('',*,*,#4620,.F.);
#5917=ORIENTED_EDGE('',*,*,#4616,.F.);
#5918=ORIENTED_EDGE('',*,*,#4621,.F.);
#5919=ORIENTED_EDGE('',*,*,#4622,.T.);
#5920=ORIENTED_EDGE('',*,*,#4623,.F.);
#5921=ORIENTED_EDGE('',*,*,#4619,.F.);
#5922=ORIENTED_EDGE('',*,*,#4624,.F.);
#5923=ORIENTED_EDGE('',*,*,#4625,.T.);
#5924=ORIENTED_EDGE('',*,*,#4626,.F.);
#5925=ORIENTED_EDGE('',*,*,#4622,.F.);
#5926=ORIENTED_EDGE('',*,*,#4627,.F.);
#5927=ORIENTED_EDGE('',*,*,#4628,.T.);
#5928=ORIENTED_EDGE('',*,*,#4629,.F.);
#5929=ORIENTED_EDGE('',*,*,#4625,.F.);
#5930=ORIENTED_EDGE('',*,*,#4630,.F.);
#5931=ORIENTED_EDGE('',*,*,#4631,.T.);
#5932=ORIENTED_EDGE('',*,*,#4632,.F.);
#5933=ORIENTED_EDGE('',*,*,#4628,.F.);
#5934=ORIENTED_EDGE('',*,*,#4633,.F.);
#5935=ORIENTED_EDGE('',*,*,#4634,.F.);
#5936=ORIENTED_EDGE('',*,*,#4635,.F.);
#5937=ORIENTED_EDGE('',*,*,#4631,.F.);
#5938=ORIENTED_EDGE('',*,*,#4636,.F.);
#5939=ORIENTED_EDGE('',*,*,#4637,.T.);
#5940=ORIENTED_EDGE('',*,*,#4638,.F.);
#5941=ORIENTED_EDGE('',*,*,#4639,.F.);
#5942=ORIENTED_EDGE('',*,*,#4640,.F.);
#5943=ORIENTED_EDGE('',*,*,#4641,.T.);
#5944=ORIENTED_EDGE('',*,*,#4642,.F.);
#5945=ORIENTED_EDGE('',*,*,#4637,.F.);
#5946=ORIENTED_EDGE('',*,*,#4643,.F.);
#5947=ORIENTED_EDGE('',*,*,#4644,.T.);
#5948=ORIENTED_EDGE('',*,*,#4645,.F.);
#5949=ORIENTED_EDGE('',*,*,#4641,.F.);
#5950=ORIENTED_EDGE('',*,*,#4646,.F.);
#5951=ORIENTED_EDGE('',*,*,#4647,.T.);
#5952=ORIENTED_EDGE('',*,*,#4648,.F.);
#5953=ORIENTED_EDGE('',*,*,#4644,.F.);
#5954=ORIENTED_EDGE('',*,*,#4649,.F.);
#5955=ORIENTED_EDGE('',*,*,#4650,.T.);
#5956=ORIENTED_EDGE('',*,*,#4651,.F.);
#5957=ORIENTED_EDGE('',*,*,#4647,.F.);
#5958=ORIENTED_EDGE('',*,*,#4652,.F.);
#5959=ORIENTED_EDGE('',*,*,#4653,.T.);
#5960=ORIENTED_EDGE('',*,*,#4654,.F.);
#5961=ORIENTED_EDGE('',*,*,#4650,.F.);
#5962=ORIENTED_EDGE('',*,*,#4655,.F.);
#5963=ORIENTED_EDGE('',*,*,#4656,.T.);
#5964=ORIENTED_EDGE('',*,*,#4657,.F.);
#5965=ORIENTED_EDGE('',*,*,#4653,.F.);
#5966=ORIENTED_EDGE('',*,*,#4658,.F.);
#5967=ORIENTED_EDGE('',*,*,#4659,.T.);
#5968=ORIENTED_EDGE('',*,*,#4660,.F.);
#5969=ORIENTED_EDGE('',*,*,#4656,.F.);
#5970=ORIENTED_EDGE('',*,*,#4661,.F.);
#5971=ORIENTED_EDGE('',*,*,#4662,.F.);
#5972=ORIENTED_EDGE('',*,*,#4663,.F.);
#5973=ORIENTED_EDGE('',*,*,#4659,.F.);
#5974=ORIENTED_EDGE('',*,*,#4664,.F.);
#5975=ORIENTED_EDGE('',*,*,#4665,.T.);
#5976=ORIENTED_EDGE('',*,*,#4666,.F.);
#5977=ORIENTED_EDGE('',*,*,#4665,.F.);
#5978=ORIENTED_EDGE('',*,*,#4578,.T.);
#5979=ORIENTED_EDGE('',*,*,#4667,.T.);
#5980=ORIENTED_EDGE('',*,*,#4668,.T.);
#5981=ORIENTED_EDGE('',*,*,#4669,.F.);
#5982=ORIENTED_EDGE('',*,*,#4555,.T.);
#5983=ORIENTED_EDGE('',*,*,#4670,.F.);
#5984=ORIENTED_EDGE('',*,*,#4671,.F.);
#5985=ORIENTED_EDGE('',*,*,#4672,.T.);
#5986=ORIENTED_EDGE('',*,*,#4606,.T.);
#5987=ORIENTED_EDGE('',*,*,#4673,.T.);
#5988=ORIENTED_EDGE('',*,*,#4671,.T.);
#5989=ORIENTED_EDGE('',*,*,#4674,.F.);
#5990=ORIENTED_EDGE('',*,*,#4583,.T.);
#5991=ORIENTED_EDGE('',*,*,#4675,.F.);
#5992=ORIENTED_EDGE('',*,*,#4676,.F.);
#5993=ORIENTED_EDGE('',*,*,#4677,.T.);
#5994=ORIENTED_EDGE('',*,*,#4634,.T.);
#5995=ORIENTED_EDGE('',*,*,#4678,.T.);
#5996=ORIENTED_EDGE('',*,*,#4676,.T.);
#5997=ORIENTED_EDGE('',*,*,#4679,.F.);
#5998=ORIENTED_EDGE('',*,*,#4611,.T.);
#5999=ORIENTED_EDGE('',*,*,#4680,.F.);
#6000=ORIENTED_EDGE('',*,*,#4681,.F.);
#6001=ORIENTED_EDGE('',*,*,#4682,.T.);
#6002=ORIENTED_EDGE('',*,*,#4662,.T.);
#6003=ORIENTED_EDGE('',*,*,#4683,.T.);
#6004=ORIENTED_EDGE('',*,*,#4681,.T.);
#6005=ORIENTED_EDGE('',*,*,#4684,.F.);
#6006=ORIENTED_EDGE('',*,*,#4639,.T.);
#6007=ORIENTED_EDGE('',*,*,#4685,.F.);
#6008=ORIENTED_EDGE('',*,*,#4668,.F.);
#6009=ORIENTED_EDGE('',*,*,#4686,.T.);
#6010=ORIENTED_EDGE('',*,*,#4554,.T.);
#6011=ORIENTED_EDGE('',*,*,#4558,.T.);
#6012=ORIENTED_EDGE('',*,*,#4561,.T.);
#6013=ORIENTED_EDGE('',*,*,#4564,.T.);
#6014=ORIENTED_EDGE('',*,*,#4567,.T.);
#6015=ORIENTED_EDGE('',*,*,#4570,.T.);
#6016=ORIENTED_EDGE('',*,*,#4573,.T.);
#6017=ORIENTED_EDGE('',*,*,#4576,.T.);
#6018=ORIENTED_EDGE('',*,*,#4579,.T.);
#6019=ORIENTED_EDGE('',*,*,#4669,.T.);
#6020=ORIENTED_EDGE('',*,*,#4685,.T.);
#6021=ORIENTED_EDGE('',*,*,#4638,.T.);
#6022=ORIENTED_EDGE('',*,*,#4642,.T.);
#6023=ORIENTED_EDGE('',*,*,#4645,.T.);
#6024=ORIENTED_EDGE('',*,*,#4648,.T.);
#6025=ORIENTED_EDGE('',*,*,#4651,.T.);
#6026=ORIENTED_EDGE('',*,*,#4654,.T.);
#6027=ORIENTED_EDGE('',*,*,#4657,.T.);
#6028=ORIENTED_EDGE('',*,*,#4660,.T.);
#6029=ORIENTED_EDGE('',*,*,#4663,.T.);
#6030=ORIENTED_EDGE('',*,*,#4684,.T.);
#6031=ORIENTED_EDGE('',*,*,#4680,.T.);
#6032=ORIENTED_EDGE('',*,*,#4610,.T.);
#6033=ORIENTED_EDGE('',*,*,#4614,.T.);
#6034=ORIENTED_EDGE('',*,*,#4617,.T.);
#6035=ORIENTED_EDGE('',*,*,#4620,.T.);
#6036=ORIENTED_EDGE('',*,*,#4623,.T.);
#6037=ORIENTED_EDGE('',*,*,#4626,.T.);
#6038=ORIENTED_EDGE('',*,*,#4629,.T.);
#6039=ORIENTED_EDGE('',*,*,#4632,.T.);
#6040=ORIENTED_EDGE('',*,*,#4635,.T.);
#6041=ORIENTED_EDGE('',*,*,#4679,.T.);
#6042=ORIENTED_EDGE('',*,*,#4675,.T.);
#6043=ORIENTED_EDGE('',*,*,#4582,.T.);
#6044=ORIENTED_EDGE('',*,*,#4586,.T.);
#6045=ORIENTED_EDGE('',*,*,#4589,.T.);
#6046=ORIENTED_EDGE('',*,*,#4592,.T.);
#6047=ORIENTED_EDGE('',*,*,#4595,.T.);
#6048=ORIENTED_EDGE('',*,*,#4598,.T.);
#6049=ORIENTED_EDGE('',*,*,#4601,.T.);
#6050=ORIENTED_EDGE('',*,*,#4604,.T.);
#6051=ORIENTED_EDGE('',*,*,#4607,.T.);
#6052=ORIENTED_EDGE('',*,*,#4674,.T.);
#6053=ORIENTED_EDGE('',*,*,#4670,.T.);
#6054=ORIENTED_EDGE('',*,*,#4666,.T.);
#6055=ORIENTED_EDGE('',*,*,#4552,.T.);
#6056=ORIENTED_EDGE('',*,*,#4672,.F.);
#6057=ORIENTED_EDGE('',*,*,#4673,.F.);
#6058=ORIENTED_EDGE('',*,*,#4605,.T.);
#6059=ORIENTED_EDGE('',*,*,#4602,.T.);
#6060=ORIENTED_EDGE('',*,*,#4599,.T.);
#6061=ORIENTED_EDGE('',*,*,#4596,.T.);
#6062=ORIENTED_EDGE('',*,*,#4593,.T.);
#6063=ORIENTED_EDGE('',*,*,#4590,.T.);
#6064=ORIENTED_EDGE('',*,*,#4587,.T.);
#6065=ORIENTED_EDGE('',*,*,#4584,.T.);
#6066=ORIENTED_EDGE('',*,*,#4580,.T.);
#6067=ORIENTED_EDGE('',*,*,#4677,.F.);
#6068=ORIENTED_EDGE('',*,*,#4678,.F.);
#6069=ORIENTED_EDGE('',*,*,#4633,.T.);
#6070=ORIENTED_EDGE('',*,*,#4630,.T.);
#6071=ORIENTED_EDGE('',*,*,#4627,.T.);
#6072=ORIENTED_EDGE('',*,*,#4624,.T.);
#6073=ORIENTED_EDGE('',*,*,#4621,.T.);
#6074=ORIENTED_EDGE('',*,*,#4618,.T.);
#6075=ORIENTED_EDGE('',*,*,#4615,.T.);
#6076=ORIENTED_EDGE('',*,*,#4612,.T.);
#6077=ORIENTED_EDGE('',*,*,#4608,.T.);
#6078=ORIENTED_EDGE('',*,*,#4682,.F.);
#6079=ORIENTED_EDGE('',*,*,#4683,.F.);
#6080=ORIENTED_EDGE('',*,*,#4661,.T.);
#6081=ORIENTED_EDGE('',*,*,#4658,.T.);
#6082=ORIENTED_EDGE('',*,*,#4655,.T.);
#6083=ORIENTED_EDGE('',*,*,#4652,.T.);
#6084=ORIENTED_EDGE('',*,*,#4649,.T.);
#6085=ORIENTED_EDGE('',*,*,#4646,.T.);
#6086=ORIENTED_EDGE('',*,*,#4643,.T.);
#6087=ORIENTED_EDGE('',*,*,#4640,.T.);
#6088=ORIENTED_EDGE('',*,*,#4636,.T.);
#6089=ORIENTED_EDGE('',*,*,#4686,.F.);
#6090=ORIENTED_EDGE('',*,*,#4667,.F.);
#6091=ORIENTED_EDGE('',*,*,#4577,.T.);
#6092=ORIENTED_EDGE('',*,*,#4574,.T.);
#6093=ORIENTED_EDGE('',*,*,#4571,.T.);
#6094=ORIENTED_EDGE('',*,*,#4568,.T.);
#6095=ORIENTED_EDGE('',*,*,#4565,.T.);
#6096=ORIENTED_EDGE('',*,*,#4562,.T.);
#6097=ORIENTED_EDGE('',*,*,#4559,.T.);
#6098=ORIENTED_EDGE('',*,*,#4556,.T.);
#6099=ORIENTED_EDGE('',*,*,#4664,.T.);
#7140=CYLINDRICAL_SURFACE('',#8214,0.21);
#7316=ADVANCED_FACE('',(#1115),#800,.F.);
#7317=ADVANCED_FACE('',(#1116),#801,.F.);
#7318=ADVANCED_FACE('',(#1117),#802,.F.);
#7319=ADVANCED_FACE('',(#1118),#803,.F.);
#7320=ADVANCED_FACE('',(#1119),#804,.F.);
#7321=ADVANCED_FACE('',(#1120),#805,.F.);
#7322=ADVANCED_FACE('',(#1121),#806,.F.);
#7323=ADVANCED_FACE('',(#1122),#807,.F.);
#7324=ADVANCED_FACE('',(#1123),#808,.F.);
#7325=ADVANCED_FACE('',(#1124),#809,.F.);
#7326=ADVANCED_FACE('',(#1125),#810,.F.);
#7327=ADVANCED_FACE('',(#1126),#811,.F.);
#7328=ADVANCED_FACE('',(#1127),#812,.F.);
#7329=ADVANCED_FACE('',(#1128),#813,.F.);
#7330=ADVANCED_FACE('',(#1129),#814,.F.);
#7331=ADVANCED_FACE('',(#1130),#815,.F.);
#7332=ADVANCED_FACE('',(#1131),#816,.F.);
#7333=ADVANCED_FACE('',(#1132),#817,.F.);
#7334=ADVANCED_FACE('',(#1133),#818,.F.);
#7335=ADVANCED_FACE('',(#1134),#819,.F.);
#7336=ADVANCED_FACE('',(#1135),#820,.F.);
#7337=ADVANCED_FACE('',(#1136),#821,.F.);
#7338=ADVANCED_FACE('',(#1137),#822,.F.);
#7339=ADVANCED_FACE('',(#1138),#823,.F.);
#7340=ADVANCED_FACE('',(#1139),#824,.F.);
#7341=ADVANCED_FACE('',(#1140),#825,.F.);
#7342=ADVANCED_FACE('',(#1141),#826,.F.);
#7343=ADVANCED_FACE('',(#1142),#827,.F.);
#7344=ADVANCED_FACE('',(#1143),#828,.F.);
#7345=ADVANCED_FACE('',(#1144),#829,.F.);
#7346=ADVANCED_FACE('',(#1145),#830,.F.);
#7347=ADVANCED_FACE('',(#1146),#831,.F.);
#7348=ADVANCED_FACE('',(#1147),#832,.F.);
#7349=ADVANCED_FACE('',(#1148),#833,.F.);
#7350=ADVANCED_FACE('',(#1149),#834,.F.);
#7351=ADVANCED_FACE('',(#1150),#835,.F.);
#7352=ADVANCED_FACE('',(#1151),#7140,.F.);
#7353=ADVANCED_FACE('',(#1152),#836,.T.);
#7354=ADVANCED_FACE('',(#1153),#837,.T.);
#7355=ADVANCED_FACE('',(#1154),#838,.T.);
#7356=ADVANCED_FACE('',(#1155),#839,.T.);
#7357=ADVANCED_FACE('',(#1156),#840,.T.);
#7358=ADVANCED_FACE('',(#1157),#841,.T.);
#7359=ADVANCED_FACE('',(#1158),#842,.T.);
#7360=ADVANCED_FACE('',(#1159),#843,.T.);
#7361=ADVANCED_FACE('',(#1160,#627),#844,.T.);
#7362=ADVANCED_FACE('',(#1161,#628),#845,.F.);
#7630=CLOSED_SHELL('',(#7316,#7317,#7318,#7319,#7320,#7321,#7322,#7323,
#7324,#7325,#7326,#7327,#7328,#7329,#7330,#7331,#7332,#7333,#7334,#7335,
#7336,#7337,#7338,#7339,#7340,#7341,#7342,#7343,#7344,#7345,#7346,#7347,
#7348,#7349,#7350,#7351,#7352,#7353,#7354,#7355,#7356,#7357,#7358,#7359,
#7360,#7361,#7362));
#8177=AXIS2_PLACEMENT_3D('',#11880,#9363,#9364);
#8178=AXIS2_PLACEMENT_3D('',#11881,#9365,#9366);
#8179=AXIS2_PLACEMENT_3D('',#11890,#9371,#9372);
#8180=AXIS2_PLACEMENT_3D('',#11896,#9376,#9377);
#8181=AXIS2_PLACEMENT_3D('',#11902,#9381,#9382);
#8182=AXIS2_PLACEMENT_3D('',#11908,#9386,#9387);
#8183=AXIS2_PLACEMENT_3D('',#11914,#9391,#9392);
#8184=AXIS2_PLACEMENT_3D('',#11920,#9396,#9397);
#8185=AXIS2_PLACEMENT_3D('',#11926,#9401,#9402);
#8186=AXIS2_PLACEMENT_3D('',#11932,#9406,#9407);
#8187=AXIS2_PLACEMENT_3D('',#11938,#9411,#9412);
#8188=AXIS2_PLACEMENT_3D('',#11947,#9417,#9418);
#8189=AXIS2_PLACEMENT_3D('',#11953,#9422,#9423);
#8190=AXIS2_PLACEMENT_3D('',#11959,#9427,#9428);
#8191=AXIS2_PLACEMENT_3D('',#11965,#9432,#9433);
#8192=AXIS2_PLACEMENT_3D('',#11971,#9437,#9438);
#8193=AXIS2_PLACEMENT_3D('',#11977,#9442,#9443);
#8194=AXIS2_PLACEMENT_3D('',#11983,#9447,#9448);
#8195=AXIS2_PLACEMENT_3D('',#11989,#9452,#9453);
#8196=AXIS2_PLACEMENT_3D('',#11995,#9457,#9458);
#8197=AXIS2_PLACEMENT_3D('',#12004,#9463,#9464);
#8198=AXIS2_PLACEMENT_3D('',#12010,#9468,#9469);
#8199=AXIS2_PLACEMENT_3D('',#12016,#9473,#9474);
#8200=AXIS2_PLACEMENT_3D('',#12022,#9478,#9479);
#8201=AXIS2_PLACEMENT_3D('',#12028,#9483,#9484);
#8202=AXIS2_PLACEMENT_3D('',#12034,#9488,#9489);
#8203=AXIS2_PLACEMENT_3D('',#12040,#9493,#9494);
#8204=AXIS2_PLACEMENT_3D('',#12046,#9498,#9499);
#8205=AXIS2_PLACEMENT_3D('',#12052,#9503,#9504);
#8206=AXIS2_PLACEMENT_3D('',#12061,#9509,#9510);
#8207=AXIS2_PLACEMENT_3D('',#12067,#9514,#9515);
#8208=AXIS2_PLACEMENT_3D('',#12073,#9519,#9520);
#8209=AXIS2_PLACEMENT_3D('',#12079,#9524,#9525);
#8210=AXIS2_PLACEMENT_3D('',#12085,#9529,#9530);
#8211=AXIS2_PLACEMENT_3D('',#12091,#9534,#9535);
#8212=AXIS2_PLACEMENT_3D('',#12097,#9539,#9540);
#8213=AXIS2_PLACEMENT_3D('',#12103,#9544,#9545);
#8214=AXIS2_PLACEMENT_3D('',#12109,#9549,#9550);
#8215=AXIS2_PLACEMENT_3D('',#12111,#9551,#9552);
#8216=AXIS2_PLACEMENT_3D('',#12114,#9554,#9555);
#8217=AXIS2_PLACEMENT_3D('',#12115,#9556,#9557);
#8218=AXIS2_PLACEMENT_3D('',#12121,#9561,#9562);
#8219=AXIS2_PLACEMENT_3D('',#12127,#9566,#9567);
#8220=AXIS2_PLACEMENT_3D('',#12130,#9570,#9571);
#8221=AXIS2_PLACEMENT_3D('',#12136,#9575,#9576);
#8222=AXIS2_PLACEMENT_3D('',#12139,#9579,#9580);
#8223=AXIS2_PLACEMENT_3D('',#12145,#9584,#9585);
#8224=AXIS2_PLACEMENT_3D('',#12148,#9588,#9589);
#8225=AXIS2_PLACEMENT_3D('',#12151,#9592,#9593);
#8226=AXIS2_PLACEMENT_3D('',#12152,#9594,#9595);
#9363=DIRECTION('axis',(0.,0.,1.));
#9364=DIRECTION('refdir',(1.,0.,0.));
#9365=DIRECTION('center_axis',(0.,0.,-1.));
#9366=DIRECTION('ref_axis',(0.,1.,0.));
#9367=DIRECTION('',(0.,1.,0.));
#9368=DIRECTION('',(1.,0.,0.));
#9369=DIRECTION('',(0.,-1.,0.));
#9370=DIRECTION('',(1.,0.,0.));
#9371=DIRECTION('center_axis',(0.,1.,-8.88178419700125E-16));
#9372=DIRECTION('ref_axis',(0.,8.88178419700125E-16,1.));
#9373=DIRECTION('',(0.,8.88178419700125E-16,1.));
#9374=DIRECTION('',(1.,0.,0.));
#9375=DIRECTION('',(0.,-8.88178419700125E-16,-1.));
#9376=DIRECTION('center_axis',(0.,-7.40148683083439E-16,-1.));
#9377=DIRECTION('ref_axis',(0.,1.,-7.40148683083439E-16));
#9378=DIRECTION('',(0.,1.,-7.40148683083439E-16));
#9379=DIRECTION('',(1.,0.,0.));
#9380=DIRECTION('',(0.,-1.,7.40148683083439E-16));
#9381=DIRECTION('center_axis',(0.,-0.707106781186547,-0.707106781186548));
#9382=DIRECTION('ref_axis',(0.,0.707106781186548,-0.707106781186547));
#9383=DIRECTION('',(0.,0.707106781186548,-0.707106781186547));
#9384=DIRECTION('',(1.,0.,0.));
#9385=DIRECTION('',(0.,-0.707106781186548,0.707106781186547));
#9386=DIRECTION('center_axis',(0.,-1.,2.77555756156289E-16));
#9387=DIRECTION('ref_axis',(0.,-2.77555756156289E-16,-1.));
#9388=DIRECTION('',(0.,-2.77555756156289E-16,-1.));
#9389=DIRECTION('',(1.,0.,0.));
#9390=DIRECTION('',(0.,2.77555756156289E-16,1.));
#9391=DIRECTION('center_axis',(0.,-0.707106781186547,0.707106781186548));
#9392=DIRECTION('ref_axis',(0.,-0.707106781186548,-0.707106781186547));
#9393=DIRECTION('',(0.,-0.707106781186548,-0.707106781186547));
#9394=DIRECTION('',(1.,0.,0.));
#9395=DIRECTION('',(0.,0.707106781186548,0.707106781186547));
#9396=DIRECTION('center_axis',(0.,7.40148683083438E-16,1.));
#9397=DIRECTION('ref_axis',(0.,-1.,7.40148683083438E-16));
#9398=DIRECTION('',(0.,-1.,7.40148683083438E-16));
#9399=DIRECTION('',(1.,0.,0.));
#9400=DIRECTION('',(0.,1.,-7.40148683083438E-16));
#9401=DIRECTION('center_axis',(0.,1.,-4.44089209850063E-16));
#9402=DIRECTION('ref_axis',(0.,4.44089209850063E-16,1.));
#9403=DIRECTION('',(0.,4.44089209850063E-16,1.));
#9404=DIRECTION('',(1.,0.,0.));
#9405=DIRECTION('',(0.,-4.44089209850063E-16,-1.));
#9406=DIRECTION('center_axis',(0.,2.41352831440251E-16,1.));
#9407=DIRECTION('ref_axis',(0.,-1.,2.41352831440251E-16));
#9408=DIRECTION('',(0.,-1.,2.41352831440251E-16));
#9409=DIRECTION('',(-1.,0.,0.));
#9410=DIRECTION('',(0.,1.,-2.41352831440251E-16));
#9411=DIRECTION('center_axis',(0.,-1.,2.41352831440251E-16));
#9412=DIRECTION('ref_axis',(0.,-2.41352831440251E-16,-1.));
#9413=DIRECTION('',(0.,-2.41352831440251E-16,-1.));
#9414=DIRECTION('',(1.,0.,0.));
#9415=DIRECTION('',(0.,2.41352831440251E-16,1.));
#9416=DIRECTION('',(1.,0.,0.));
#9417=DIRECTION('center_axis',(0.,0.,-1.));
#9418=DIRECTION('ref_axis',(0.,1.,0.));
#9419=DIRECTION('',(0.,1.,0.));
#9420=DIRECTION('',(1.,0.,0.));
#9421=DIRECTION('',(0.,-1.,0.));
#9422=DIRECTION('center_axis',(0.,-1.,0.));
#9423=DIRECTION('ref_axis',(0.,0.,-1.));
#9424=DIRECTION('',(0.,0.,-1.));
#9425=DIRECTION('',(1.,0.,0.));
#9426=DIRECTION('',(0.,0.,1.));
#9427=DIRECTION('center_axis',(0.,-0.707106781186547,0.707106781186548));
#9428=DIRECTION('ref_axis',(0.,-0.707106781186548,-0.707106781186547));
#9429=DIRECTION('',(0.,-0.707106781186548,-0.707106781186547));
#9430=DIRECTION('',(1.,0.,0.));
#9431=DIRECTION('',(0.,0.707106781186548,0.707106781186547));
#9432=DIRECTION('center_axis',(0.,0.,1.));
#9433=DIRECTION('ref_axis',(0.,-1.,0.));
#9434=DIRECTION('',(0.,-1.,0.));
#9435=DIRECTION('',(1.,0.,0.));
#9436=DIRECTION('',(0.,1.,0.));
#9437=DIRECTION('center_axis',(0.,0.707106781186548,0.707106781186547));
#9438=DIRECTION('ref_axis',(0.,-0.707106781186547,0.707106781186548));
#9439=DIRECTION('',(0.,-0.707106781186547,0.707106781186548));
#9440=DIRECTION('',(1.,0.,0.));
#9441=DIRECTION('',(0.,0.707106781186547,-0.707106781186548));
#9442=DIRECTION('center_axis',(0.,1.,0.));
#9443=DIRECTION('ref_axis',(0.,0.,1.));
#9444=DIRECTION('',(0.,0.,1.));
#9445=DIRECTION('',(1.,0.,0.));
#9446=DIRECTION('',(0.,0.,-1.));
#9447=DIRECTION('center_axis',(0.,0.,-1.));
#9448=DIRECTION('ref_axis',(0.,1.,0.));
#9449=DIRECTION('',(0.,1.,0.));
#9450=DIRECTION('',(1.,0.,0.));
#9451=DIRECTION('',(0.,-1.,0.));
#9452=DIRECTION('center_axis',(0.,1.,-2.41352831440251E-16));
#9453=DIRECTION('ref_axis',(0.,2.41352831440251E-16,1.));
#9454=DIRECTION('',(0.,2.41352831440251E-16,1.));
#9455=DIRECTION('',(-1.,0.,0.));
#9456=DIRECTION('',(0.,-2.41352831440251E-16,-1.));
#9457=DIRECTION('center_axis',(0.,0.,1.));
#9458=DIRECTION('ref_axis',(0.,-1.,0.));
#9459=DIRECTION('',(0.,-1.,0.));
#9460=DIRECTION('',(1.,0.,0.));
#9461=DIRECTION('',(0.,1.,0.));
#9462=DIRECTION('',(1.,0.,0.));
#9463=DIRECTION('center_axis',(0.,-1.,0.));
#9464=DIRECTION('ref_axis',(0.,0.,-1.));
#9465=DIRECTION('',(0.,0.,-1.));
#9466=DIRECTION('',(1.,0.,0.));
#9467=DIRECTION('',(0.,0.,1.));
#9468=DIRECTION('center_axis',(0.,0.,1.));
#9469=DIRECTION('ref_axis',(0.,-1.,0.));
#9470=DIRECTION('',(0.,-1.,0.));
#9471=DIRECTION('',(1.,0.,0.));
#9472=DIRECTION('',(0.,1.,0.));
#9473=DIRECTION('center_axis',(0.,0.707106781186548,0.707106781186548));
#9474=DIRECTION('ref_axis',(0.,-0.707106781186548,0.707106781186548));
#9475=DIRECTION('',(0.,-0.707106781186548,0.707106781186548));
#9476=DIRECTION('',(1.,0.,0.));
#9477=DIRECTION('',(0.,0.707106781186548,-0.707106781186548));
#9478=DIRECTION('center_axis',(0.,1.,0.));
#9479=DIRECTION('ref_axis',(0.,0.,1.));
#9480=DIRECTION('',(0.,0.,1.));
#9481=DIRECTION('',(1.,0.,0.));
#9482=DIRECTION('',(0.,0.,-1.));
#9483=DIRECTION('center_axis',(0.,0.707106781186548,-0.707106781186547));
#9484=DIRECTION('ref_axis',(0.,0.707106781186547,0.707106781186548));
#9485=DIRECTION('',(0.,0.707106781186547,0.707106781186548));
#9486=DIRECTION('',(1.,0.,0.));
#9487=DIRECTION('',(0.,-0.707106781186547,-0.707106781186548));
#9488=DIRECTION('center_axis',(0.,-7.40148683083438E-16,-1.));
#9489=DIRECTION('ref_axis',(0.,1.,-7.40148683083438E-16));
#9490=DIRECTION('',(0.,1.,-7.40148683083438E-16));
#9491=DIRECTION('',(1.,0.,0.));
#9492=DIRECTION('',(0.,-1.,7.40148683083438E-16));
#9493=DIRECTION('center_axis',(0.,-1.,0.));
#9494=DIRECTION('ref_axis',(0.,0.,-1.));
#9495=DIRECTION('',(0.,0.,-1.));
#9496=DIRECTION('',(1.,0.,0.));
#9497=DIRECTION('',(0.,0.,1.));
#9498=DIRECTION('center_axis',(0.,0.,-1.));
#9499=DIRECTION('ref_axis',(0.,1.,0.));
#9500=DIRECTION('',(0.,1.,0.));
#9501=DIRECTION('',(-1.,0.,0.));
#9502=DIRECTION('',(0.,-1.,0.));
#9503=DIRECTION('center_axis',(0.,1.,0.));
#9504=DIRECTION('ref_axis',(0.,0.,1.));
#9505=DIRECTION('',(0.,0.,1.));
#9506=DIRECTION('',(1.,0.,0.));
#9507=DIRECTION('',(0.,0.,-1.));
#9508=DIRECTION('',(1.,0.,0.));
#9509=DIRECTION('center_axis',(0.,0.,1.));
#9510=DIRECTION('ref_axis',(0.,-1.,0.));
#9511=DIRECTION('',(0.,-1.,0.));
#9512=DIRECTION('',(1.,0.,0.));
#9513=DIRECTION('',(0.,1.,0.));
#9514=DIRECTION('center_axis',(0.,1.,0.));
#9515=DIRECTION('ref_axis',(0.,0.,1.));
#9516=DIRECTION('',(0.,0.,1.));
#9517=DIRECTION('',(1.,0.,0.));
#9518=DIRECTION('',(0.,0.,-1.));
#9519=DIRECTION('center_axis',(0.,0.707106781186547,-0.707106781186548));
#9520=DIRECTION('ref_axis',(0.,0.707106781186548,0.707106781186547));
#9521=DIRECTION('',(0.,0.707106781186548,0.707106781186547));
#9522=DIRECTION('',(1.,0.,0.));
#9523=DIRECTION('',(0.,-0.707106781186548,-0.707106781186547));
#9524=DIRECTION('center_axis',(0.,0.,-1.));
#9525=DIRECTION('ref_axis',(0.,1.,0.));
#9526=DIRECTION('',(0.,1.,0.));
#9527=DIRECTION('',(1.,0.,0.));
#9528=DIRECTION('',(0.,-1.,0.));
#9529=DIRECTION('center_axis',(0.,-0.707106781186547,-0.707106781186548));
#9530=DIRECTION('ref_axis',(0.,0.707106781186548,-0.707106781186547));
#9531=DIRECTION('',(0.,0.707106781186548,-0.707106781186547));
#9532=DIRECTION('',(1.,0.,0.));
#9533=DIRECTION('',(0.,-0.707106781186548,0.707106781186547));
#9534=DIRECTION('center_axis',(0.,-1.,0.));
#9535=DIRECTION('ref_axis',(0.,0.,-1.));
#9536=DIRECTION('',(0.,0.,-1.));
#9537=DIRECTION('',(1.,0.,0.));
#9538=DIRECTION('',(0.,0.,1.));
#9539=DIRECTION('center_axis',(0.,0.,1.));
#9540=DIRECTION('ref_axis',(0.,-1.,0.));
#9541=DIRECTION('',(0.,-1.,0.));
#9542=DIRECTION('',(1.,0.,0.));
#9543=DIRECTION('',(0.,1.,0.));
#9544=DIRECTION('center_axis',(0.,-1.,0.));
#9545=DIRECTION('ref_axis',(0.,0.,-1.));
#9546=DIRECTION('',(0.,0.,-1.));
#9547=DIRECTION('',(-1.,0.,0.));
#9548=DIRECTION('',(0.,0.,1.));
#9549=DIRECTION('center_axis',(1.,0.,0.));
#9550=DIRECTION('ref_axis',(0.,0.,-1.));
#9551=DIRECTION('center_axis',(1.,0.,0.));
#9552=DIRECTION('ref_axis',(0.,0.,-1.));
#9553=DIRECTION('',(1.,0.,0.));
#9554=DIRECTION('center_axis',(-1.,0.,0.));
#9555=DIRECTION('ref_axis',(0.,0.,-1.));
#9556=DIRECTION('center_axis',(0.,1.,0.));
#9557=DIRECTION('ref_axis',(0.,0.,1.));
#9558=DIRECTION('',(0.,0.,1.));
#9559=DIRECTION('',(1.,0.,0.));
#9560=DIRECTION('',(0.,0.,1.));
#9561=DIRECTION('center_axis',(0.,1.,0.));
#9562=DIRECTION('ref_axis',(0.,0.,1.));
#9563=DIRECTION('',(0.,0.,1.));
#9564=DIRECTION('',(1.,0.,0.));
#9565=DIRECTION('',(0.,0.,1.));
#9566=DIRECTION('center_axis',(0.,0.,-1.));
#9567=DIRECTION('ref_axis',(0.,1.,0.));
#9568=DIRECTION('',(0.,1.,0.));
#9569=DIRECTION('',(0.,1.,0.));
#9570=DIRECTION('center_axis',(0.,0.,-1.));
#9571=DIRECTION('ref_axis',(0.,1.,0.));
#9572=DIRECTION('',(0.,1.,0.));
#9573=DIRECTION('',(1.,0.,0.));
#9574=DIRECTION('',(0.,1.,0.));
#9575=DIRECTION('center_axis',(0.,-1.,0.));
#9576=DIRECTION('ref_axis',(0.,0.,-1.));
#9577=DIRECTION('',(0.,0.,-1.));
#9578=DIRECTION('',(0.,0.,-1.));
#9579=DIRECTION('center_axis',(0.,-1.,0.));
#9580=DIRECTION('ref_axis',(0.,0.,-1.));
#9581=DIRECTION('',(0.,0.,-1.));
#9582=DIRECTION('',(1.,0.,0.));
#9583=DIRECTION('',(0.,0.,-1.));
#9584=DIRECTION('center_axis',(0.,0.,1.));
#9585=DIRECTION('ref_axis',(0.,-1.,0.));
#9586=DIRECTION('',(0.,-1.,0.));
#9587=DIRECTION('',(0.,-1.,0.));
#9588=DIRECTION('center_axis',(0.,0.,1.));
#9589=DIRECTION('ref_axis',(0.,-1.,0.));
#9590=DIRECTION('',(0.,-1.,0.));
#9591=DIRECTION('',(0.,-1.,0.));
#9592=DIRECTION('center_axis',(1.,0.,0.));
#9593=DIRECTION('ref_axis',(0.,0.,-1.));
#9594=DIRECTION('center_axis',(1.,0.,0.));
#9595=DIRECTION('ref_axis',(0.,0.,-1.));
#11880=CARTESIAN_POINT('',(0.,0.,0.));
#11881=CARTESIAN_POINT('Origin',(-0.1,0.82,-0.3));
#11882=CARTESIAN_POINT('',(0.,0.82,-0.3));
#11883=CARTESIAN_POINT('',(0.,1.,-0.3));
#11884=CARTESIAN_POINT('',(0.,0.41,-0.3));
#11885=CARTESIAN_POINT('',(20.,0.82,-0.3));
#11886=CARTESIAN_POINT('',(-0.1,0.82,-0.3));
#11887=CARTESIAN_POINT('',(20.,1.,-0.3));
#11888=CARTESIAN_POINT('',(20.,0.41,-0.3));
#11889=CARTESIAN_POINT('',(-0.05,1.,-0.3));
#11890=CARTESIAN_POINT('Origin',(-0.1,0.82,-0.55));
#11891=CARTESIAN_POINT('',(0.,0.82,-0.55));
#11892=CARTESIAN_POINT('',(0.,0.82,-0.275));
#11893=CARTESIAN_POINT('',(20.,0.82,-0.55));
#11894=CARTESIAN_POINT('',(-0.1,0.82,-0.55));
#11895=CARTESIAN_POINT('',(20.,0.82,-0.275));
#11896=CARTESIAN_POINT('Origin',(-0.1,0.67,-0.55));
#11897=CARTESIAN_POINT('',(0.,0.67,-0.55));
#11898=CARTESIAN_POINT('',(0.,0.335,-0.55));
#11899=CARTESIAN_POINT('',(20.,0.67,-0.55));
#11900=CARTESIAN_POINT('',(-0.1,0.67,-0.55));
#11901=CARTESIAN_POINT('',(20.,0.335,-0.55));
#11902=CARTESIAN_POINT('Origin',(-0.1,0.42,-0.3));
#11903=CARTESIAN_POINT('',(0.,0.42,-0.3));
#11904=CARTESIAN_POINT('',(0.,0.24,-0.12));
#11905=CARTESIAN_POINT('',(20.,0.42,-0.3));
#11906=CARTESIAN_POINT('',(-0.1,0.42,-0.3));
#11907=CARTESIAN_POINT('',(20.,0.24,-0.12));
#11908=CARTESIAN_POINT('Origin',(-0.1,0.42,0.3));
#11909=CARTESIAN_POINT('',(0.,0.42,0.3));
#11910=CARTESIAN_POINT('',(0.,0.42,0.15));
#11911=CARTESIAN_POINT('',(20.,0.42,0.3));
#11912=CARTESIAN_POINT('',(-0.1,0.42,0.3));
#11913=CARTESIAN_POINT('',(20.,0.42,0.15));
#11914=CARTESIAN_POINT('Origin',(-0.1,0.67,0.55));
#11915=CARTESIAN_POINT('',(0.,0.67,0.55));
#11916=CARTESIAN_POINT('',(6.93889390390723E-18,0.365,0.245));
#11917=CARTESIAN_POINT('',(20.,0.67,0.55));
#11918=CARTESIAN_POINT('',(-0.1,0.67,0.55));
#11919=CARTESIAN_POINT('',(20.,0.365,0.245));
#11920=CARTESIAN_POINT('Origin',(-0.1,0.82,0.55));
#11921=CARTESIAN_POINT('',(0.,0.82,0.55));
#11922=CARTESIAN_POINT('',(0.,0.41,0.55));
#11923=CARTESIAN_POINT('',(20.,0.82,0.55));
#11924=CARTESIAN_POINT('',(-0.1,0.82,0.55));
#11925=CARTESIAN_POINT('',(20.,0.41,0.55));
#11926=CARTESIAN_POINT('Origin',(-0.1,0.82,0.3));
#11927=CARTESIAN_POINT('',(0.,0.82,0.3));
#11928=CARTESIAN_POINT('',(0.,0.82,0.15));
#11929=CARTESIAN_POINT('',(20.,0.82,0.3));
#11930=CARTESIAN_POINT('',(-0.1,0.82,0.3));
#11931=CARTESIAN_POINT('',(20.,0.82,0.15));
#11932=CARTESIAN_POINT('Origin',(-0.1,1.05,0.3));
#11933=CARTESIAN_POINT('',(0.,1.,0.3));
#11934=CARTESIAN_POINT('',(0.,0.525,0.3));
#11935=CARTESIAN_POINT('',(20.,1.,0.3));
#11936=CARTESIAN_POINT('',(-0.05,1.,0.3));
#11937=CARTESIAN_POINT('',(20.,0.525,0.3));
#11938=CARTESIAN_POINT('Origin',(-0.1,-0.3,-0.82));
#11939=CARTESIAN_POINT('',(0.,-0.3,-0.82));
#11940=CARTESIAN_POINT('',(0.,-0.3,-1.));
#11941=CARTESIAN_POINT('',(0.,-0.3,-0.41));
#11942=CARTESIAN_POINT('',(20.,-0.3,-0.82));
#11943=CARTESIAN_POINT('',(-0.1,-0.3,-0.82));
#11944=CARTESIAN_POINT('',(20.,-0.3,-1.));
#11945=CARTESIAN_POINT('',(20.,-0.3,-0.41));
#11946=CARTESIAN_POINT('',(-0.05,-0.3,-1.));
#11947=CARTESIAN_POINT('Origin',(-0.1,-0.55,-0.82));
#11948=CARTESIAN_POINT('',(0.,-0.55,-0.82));
#11949=CARTESIAN_POINT('',(0.,-0.275,-0.82));
#11950=CARTESIAN_POINT('',(20.,-0.55,-0.82));
#11951=CARTESIAN_POINT('',(-0.1,-0.55,-0.82));
#11952=CARTESIAN_POINT('',(20.,-0.275,-0.82));
#11953=CARTESIAN_POINT('Origin',(-0.1,-0.55,-0.67));
#11954=CARTESIAN_POINT('',(0.,-0.55,-0.67));
#11955=CARTESIAN_POINT('',(0.,-0.55,-0.335));
#11956=CARTESIAN_POINT('',(20.,-0.55,-0.67));
#11957=CARTESIAN_POINT('',(-0.1,-0.55,-0.67));
#11958=CARTESIAN_POINT('',(20.,-0.55,-0.335));
#11959=CARTESIAN_POINT('Origin',(-0.1,-0.3,-0.42));
#11960=CARTESIAN_POINT('',(0.,-0.3,-0.42));
#11961=CARTESIAN_POINT('',(0.,-0.12,-0.24));
#11962=CARTESIAN_POINT('',(20.,-0.3,-0.42));
#11963=CARTESIAN_POINT('',(-0.1,-0.3,-0.42));
#11964=CARTESIAN_POINT('',(20.,-0.12,-0.24));
#11965=CARTESIAN_POINT('Origin',(-0.1,0.3,-0.42));
#11966=CARTESIAN_POINT('',(0.,0.3,-0.42));
#11967=CARTESIAN_POINT('',(0.,0.15,-0.42));
#11968=CARTESIAN_POINT('',(20.,0.3,-0.42));
#11969=CARTESIAN_POINT('',(-0.1,0.3,-0.42));
#11970=CARTESIAN_POINT('',(20.,0.15,-0.42));
#11971=CARTESIAN_POINT('Origin',(-0.1,0.55,-0.67));
#11972=CARTESIAN_POINT('',(0.,0.55,-0.67));
#11973=CARTESIAN_POINT('',(0.,0.245,-0.365));
#11974=CARTESIAN_POINT('',(20.,0.55,-0.67));
#11975=CARTESIAN_POINT('',(-0.1,0.55,-0.67));
#11976=CARTESIAN_POINT('',(20.,0.245,-0.365));
#11977=CARTESIAN_POINT('Origin',(-0.1,0.55,-0.82));
#11978=CARTESIAN_POINT('',(0.,0.55,-0.82));
#11979=CARTESIAN_POINT('',(0.,0.55,-0.41));
#11980=CARTESIAN_POINT('',(20.,0.55,-0.82));
#11981=CARTESIAN_POINT('',(-0.1,0.55,-0.82));
#11982=CARTESIAN_POINT('',(20.,0.55,-0.41));
#11983=CARTESIAN_POINT('Origin',(-0.1,0.3,-0.82));
#11984=CARTESIAN_POINT('',(0.,0.3,-0.82));
#11985=CARTESIAN_POINT('',(0.,0.15,-0.82));
#11986=CARTESIAN_POINT('',(20.,0.3,-0.82));
#11987=CARTESIAN_POINT('',(-0.1,0.3,-0.82));
#11988=CARTESIAN_POINT('',(20.,0.15,-0.82));
#11989=CARTESIAN_POINT('Origin',(-0.1,0.3,-1.05));
#11990=CARTESIAN_POINT('',(0.,0.3,-1.));
#11991=CARTESIAN_POINT('',(0.,0.3,-0.525));
#11992=CARTESIAN_POINT('',(20.,0.3,-1.));
#11993=CARTESIAN_POINT('',(-0.05,0.3,-1.));
#11994=CARTESIAN_POINT('',(20.,0.3,-0.525));
#11995=CARTESIAN_POINT('Origin',(-0.1,-0.82,0.3));
#11996=CARTESIAN_POINT('',(0.,-0.82,0.3));
#11997=CARTESIAN_POINT('',(0.,-1.,0.3));
#11998=CARTESIAN_POINT('',(0.,-0.41,0.3));
#11999=CARTESIAN_POINT('',(20.,-0.82,0.3));
#12000=CARTESIAN_POINT('',(-0.1,-0.82,0.3));
#12001=CARTESIAN_POINT('',(20.,-1.,0.3));
#12002=CARTESIAN_POINT('',(20.,-0.41,0.3));
#12003=CARTESIAN_POINT('',(-0.05,-1.,0.3));
#12004=CARTESIAN_POINT('Origin',(-0.1,-0.82,0.55));
#12005=CARTESIAN_POINT('',(0.,-0.82,0.55));
#12006=CARTESIAN_POINT('',(0.,-0.82,0.275));
#12007=CARTESIAN_POINT('',(20.,-0.82,0.55));
#12008=CARTESIAN_POINT('',(-0.1,-0.82,0.55));
#12009=CARTESIAN_POINT('',(20.,-0.82,0.275));
#12010=CARTESIAN_POINT('Origin',(-0.1,-0.67,0.55));
#12011=CARTESIAN_POINT('',(0.,-0.67,0.55));
#12012=CARTESIAN_POINT('',(0.,-0.335,0.55));
#12013=CARTESIAN_POINT('',(20.,-0.67,0.55));
#12014=CARTESIAN_POINT('',(-0.1,-0.67,0.55));
#12015=CARTESIAN_POINT('',(20.,-0.335,0.55));
#12016=CARTESIAN_POINT('Origin',(-0.1,-0.42,0.3));
#12017=CARTESIAN_POINT('',(0.,-0.42,0.3));
#12018=CARTESIAN_POINT('',(-6.93889390390723E-18,-0.24,0.12));
#12019=CARTESIAN_POINT('',(20.,-0.42,0.3));
#12020=CARTESIAN_POINT('',(-0.1,-0.42,0.3));
#12021=CARTESIAN_POINT('',(20.,-0.24,0.12));
#12022=CARTESIAN_POINT('Origin',(-0.1,-0.42,-0.3));
#12023=CARTESIAN_POINT('',(0.,-0.42,-0.3));
#12024=CARTESIAN_POINT('',(0.,-0.42,-0.15));
#12025=CARTESIAN_POINT('',(20.,-0.42,-0.3));
#12026=CARTESIAN_POINT('',(-0.1,-0.42,-0.3));
#12027=CARTESIAN_POINT('',(20.,-0.42,-0.15));
#12028=CARTESIAN_POINT('Origin',(-0.1,-0.67,-0.55));
#12029=CARTESIAN_POINT('',(0.,-0.67,-0.55));
#12030=CARTESIAN_POINT('',(0.,-0.365,-0.245));
#12031=CARTESIAN_POINT('',(20.,-0.67,-0.55));
#12032=CARTESIAN_POINT('',(-0.1,-0.67,-0.55));
#12033=CARTESIAN_POINT('',(20.,-0.365,-0.245));
#12034=CARTESIAN_POINT('Origin',(-0.1,-0.82,-0.55));
#12035=CARTESIAN_POINT('',(0.,-0.82,-0.55));
#12036=CARTESIAN_POINT('',(0.,-0.41,-0.55));
#12037=CARTESIAN_POINT('',(20.,-0.82,-0.55));
#12038=CARTESIAN_POINT('',(-0.1,-0.82,-0.55));
#12039=CARTESIAN_POINT('',(20.,-0.41,-0.55));
#12040=CARTESIAN_POINT('Origin',(-0.1,-0.82,-0.3));
#12041=CARTESIAN_POINT('',(0.,-0.82,-0.3));
#12042=CARTESIAN_POINT('',(0.,-0.82,-0.15));
#12043=CARTESIAN_POINT('',(20.,-0.82,-0.3));
#12044=CARTESIAN_POINT('',(-0.1,-0.82,-0.3));
#12045=CARTESIAN_POINT('',(20.,-0.82,-0.15));
#12046=CARTESIAN_POINT('Origin',(-0.1,-1.05,-0.3));
#12047=CARTESIAN_POINT('',(0.,-1.,-0.3));
#12048=CARTESIAN_POINT('',(0.,-0.525,-0.3));
#12049=CARTESIAN_POINT('',(20.,-1.,-0.3));
#12050=CARTESIAN_POINT('',(-0.05,-1.,-0.3));
#12051=CARTESIAN_POINT('',(20.,-0.525,-0.3));
#12052=CARTESIAN_POINT('Origin',(-0.1,0.3,0.82));
#12053=CARTESIAN_POINT('',(0.,0.3,0.82));
#12054=CARTESIAN_POINT('',(0.,0.3,1.));
#12055=CARTESIAN_POINT('',(0.,0.3,0.41));
#12056=CARTESIAN_POINT('',(20.,0.3,0.82));
#12057=CARTESIAN_POINT('',(-0.1,0.3,0.82));
#12058=CARTESIAN_POINT('',(20.,0.3,1.));
#12059=CARTESIAN_POINT('',(20.,0.3,0.41));
#12060=CARTESIAN_POINT('',(-0.05,0.3,1.));
#12061=CARTESIAN_POINT('Origin',(-0.1,0.55,0.82));
#12062=CARTESIAN_POINT('',(0.,0.55,0.82));
#12063=CARTESIAN_POINT('',(0.,0.275,0.82));
#12064=CARTESIAN_POINT('',(20.,0.55,0.82));
#12065=CARTESIAN_POINT('',(-0.1,0.55,0.82));
#12066=CARTESIAN_POINT('',(20.,0.275,0.82));
#12067=CARTESIAN_POINT('Origin',(-0.1,0.55,0.67));
#12068=CARTESIAN_POINT('',(0.,0.55,0.67));
#12069=CARTESIAN_POINT('',(0.,0.55,0.335));
#12070=CARTESIAN_POINT('',(20.,0.55,0.67));
#12071=CARTESIAN_POINT('',(-0.1,0.55,0.67));
#12072=CARTESIAN_POINT('',(20.,0.55,0.335));
#12073=CARTESIAN_POINT('Origin',(-0.1,0.3,0.42));
#12074=CARTESIAN_POINT('',(0.,0.3,0.42));
#12075=CARTESIAN_POINT('',(6.93889390390723E-18,0.12,0.24));
#12076=CARTESIAN_POINT('',(20.,0.3,0.42));
#12077=CARTESIAN_POINT('',(-0.1,0.3,0.42));
#12078=CARTESIAN_POINT('',(20.,0.12,0.24));
#12079=CARTESIAN_POINT('Origin',(-0.1,-0.3,0.42));
#12080=CARTESIAN_POINT('',(0.,-0.3,0.42));
#12081=CARTESIAN_POINT('',(0.,-0.15,0.42));
#12082=CARTESIAN_POINT('',(20.,-0.3,0.42));
#12083=CARTESIAN_POINT('',(-0.1,-0.3,0.42));
#12084=CARTESIAN_POINT('',(20.,-0.15,0.42));
#12085=CARTESIAN_POINT('Origin',(-0.1,-0.55,0.67));
#12086=CARTESIAN_POINT('',(0.,-0.55,0.67));
#12087=CARTESIAN_POINT('',(6.93889390390723E-18,-0.245,0.365));
#12088=CARTESIAN_POINT('',(20.,-0.55,0.67));
#12089=CARTESIAN_POINT('',(-0.1,-0.55,0.67));
#12090=CARTESIAN_POINT('',(20.,-0.245,0.365));
#12091=CARTESIAN_POINT('Origin',(-0.1,-0.55,0.82));
#12092=CARTESIAN_POINT('',(0.,-0.55,0.82));
#12093=CARTESIAN_POINT('',(0.,-0.55,0.41));
#12094=CARTESIAN_POINT('',(20.,-0.55,0.82));
#12095=CARTESIAN_POINT('',(-0.1,-0.55,0.82));
#12096=CARTESIAN_POINT('',(20.,-0.55,0.41));
#12097=CARTESIAN_POINT('Origin',(-0.1,-0.3,0.82));
#12098=CARTESIAN_POINT('',(0.,-0.3,0.82));
#12099=CARTESIAN_POINT('',(0.,-0.15,0.82));
#12100=CARTESIAN_POINT('',(20.,-0.3,0.82));
#12101=CARTESIAN_POINT('',(-0.1,-0.3,0.82));
#12102=CARTESIAN_POINT('',(20.,-0.15,0.82));
#12103=CARTESIAN_POINT('Origin',(-0.1,-0.3,1.05));
#12104=CARTESIAN_POINT('',(0.,-0.3,1.));
#12105=CARTESIAN_POINT('',(0.,-0.3,0.525));
#12106=CARTESIAN_POINT('',(20.,-0.3,1.));
#12107=CARTESIAN_POINT('',(-0.05,-0.3,1.));
#12108=CARTESIAN_POINT('',(20.,-0.3,0.525));
#12109=CARTESIAN_POINT('Origin',(-0.1,0.,0.));
#12110=CARTESIAN_POINT('',(0.,-2.57175827820944E-17,0.21));
#12111=CARTESIAN_POINT('Origin',(0.,0.,0.));
#12112=CARTESIAN_POINT('',(20.,2.57175827820944E-17,0.21));
#12113=CARTESIAN_POINT('',(-0.1,-2.57175827820944E-17,0.21));
#12114=CARTESIAN_POINT('Origin',(20.,0.,0.));
#12115=CARTESIAN_POINT('Origin',(0.,1.,-1.));
#12116=CARTESIAN_POINT('',(0.,1.,1.));
#12117=CARTESIAN_POINT('',(0.,1.,-1.));
#12118=CARTESIAN_POINT('',(20.,1.,1.));
#12119=CARTESIAN_POINT('',(0.,1.,1.));
#12120=CARTESIAN_POINT('',(20.,1.,-1.));
#12121=CARTESIAN_POINT('Origin',(0.,1.,-1.));
#12122=CARTESIAN_POINT('',(20.,1.,-1.));
#12123=CARTESIAN_POINT('',(20.,1.,-1.));
#12124=CARTESIAN_POINT('',(0.,1.,-1.));
#12125=CARTESIAN_POINT('',(0.,1.,-1.));
#12126=CARTESIAN_POINT('',(0.,1.,-1.));
#12127=CARTESIAN_POINT('Origin',(0.,-1.,-1.));
#12128=CARTESIAN_POINT('',(0.,-1.,-1.));
#12129=CARTESIAN_POINT('',(20.,-1.,-1.));
#12130=CARTESIAN_POINT('Origin',(0.,-1.,-1.));
#12131=CARTESIAN_POINT('',(20.,-1.,-1.));
#12132=CARTESIAN_POINT('',(20.,-1.,-1.));
#12133=CARTESIAN_POINT('',(0.,-1.,-1.));
#12134=CARTESIAN_POINT('',(0.,-1.,-1.));
#12135=CARTESIAN_POINT('',(0.,-1.,-1.));
#12136=CARTESIAN_POINT('Origin',(0.,-1.,1.));
#12137=CARTESIAN_POINT('',(0.,-1.,1.));
#12138=CARTESIAN_POINT('',(20.,-1.,1.));
#12139=CARTESIAN_POINT('Origin',(0.,-1.,1.));
#12140=CARTESIAN_POINT('',(20.,-1.,1.));
#12141=CARTESIAN_POINT('',(20.,-1.,1.));
#12142=CARTESIAN_POINT('',(0.,-1.,1.));
#12143=CARTESIAN_POINT('',(0.,-1.,1.));
#12144=CARTESIAN_POINT('',(0.,-1.,1.));
#12145=CARTESIAN_POINT('Origin',(0.,1.,1.));
#12146=CARTESIAN_POINT('',(0.,1.,1.));
#12147=CARTESIAN_POINT('',(20.,1.,1.));
#12148=CARTESIAN_POINT('Origin',(0.,1.,1.));
#12149=CARTESIAN_POINT('',(20.,1.,1.));
#12150=CARTESIAN_POINT('',(0.,1.,1.));
#12151=CARTESIAN_POINT('Origin',(20.,0.,0.));
#12152=CARTESIAN_POINT('Origin',(0.,0.,0.));
#13749=UNCERTAINTY_MEASURE_WITH_UNIT(LENGTH_MEASURE(0.001),#13822,
'DISTANCE_ACCURACY_VALUE',
'Maximum model space distance between geometric entities at asserted c
onnectivities');
#13782=UNCERTAINTY_MEASURE_WITH_UNIT(LENGTH_MEASURE(0.001),#13822,
'DISTANCE_ACCURACY_VALUE',
'Maximum model space distance between geometric entities at asserted c
onnectivities');
#13788=(
GEOMETRIC_REPRESENTATION_CONTEXT(3)
GLOBAL_UNCERTAINTY_ASSIGNED_CONTEXT((#13749))
GLOBAL_UNIT_ASSIGNED_CONTEXT((#13822,#13824,#13825))
REPRESENTATION_CONTEXT('','3D')
);
#13821=(
GEOMETRIC_REPRESENTATION_CONTEXT(3)
GLOBAL_UNCERTAINTY_ASSIGNED_CONTEXT((#13782))
GLOBAL_UNIT_ASSIGNED_CONTEXT((#13822,#13824,#13825))
REPRESENTATION_CONTEXT('','3D')
);
#13822=(
LENGTH_UNIT()
NAMED_UNIT(*)
SI_UNIT(.CENTI.,.METRE.)
);
#13824=(
NAMED_UNIT(*)
PLANE_ANGLE_UNIT()
SI_UNIT($,.RADIAN.)
);
#13825=(
NAMED_UNIT(*)
SI_UNIT($,.STERADIAN.)
SOLID_ANGLE_UNIT()
);
#13831=SHAPE_DEFINITION_REPRESENTATION(#13869,#14001);
#13869=PRODUCT_DEFINITION_SHAPE('',$,#14040);
#14001=SHAPE_REPRESENTATION('',(#8177),#13788);
#14034=PRODUCT_DEFINITION_CONTEXT('part definition',#14150,'design');
#14040=PRODUCT_DEFINITION('Slotted Extrusion - 20 x 20 x 200 mm',
'Slotted Extrusion - 20 x 20 x 200 mm',#14078,#14034);
#14078=PRODUCT_DEFINITION_FORMATION('',$,#14157);
#14150=APPLICATION_CONTEXT(
'Core Data for Automotive Mechanical Design Process');
#14151=PRODUCT_CONTEXT('part definition',#14150,'mechanical');
#14157=PRODUCT('Slotted Extrusion - 20 x 20 x 200 mm',
'Slotted Extrusion - 20 x 20 x 200 mm',
'Slotted Extrusion - 20 x 20 x 200 mm',(#14151));
#14192=PRESENTATION_STYLE_ASSIGNMENT((#14197));
#14197=SURFACE_STYLE_USAGE(.BOTH.,#14202);
#14202=SURFACE_SIDE_STYLE('',(#14207));
#14207=SURFACE_STYLE_FILL_AREA(#14212);
#14212=FILL_AREA_STYLE('CAD Library Painted - Engineering blue',(#14217));
#14217=FILL_AREA_STYLE_COLOUR('CAD Library Painted - Engineering blue',
#14222);
#14222=COLOUR_RGB('CAD Library Painted - Engineering blue',0.12156862745098,
0.356862745098039,0.6);
ENDSEC;
END-ISO-10303-21;
